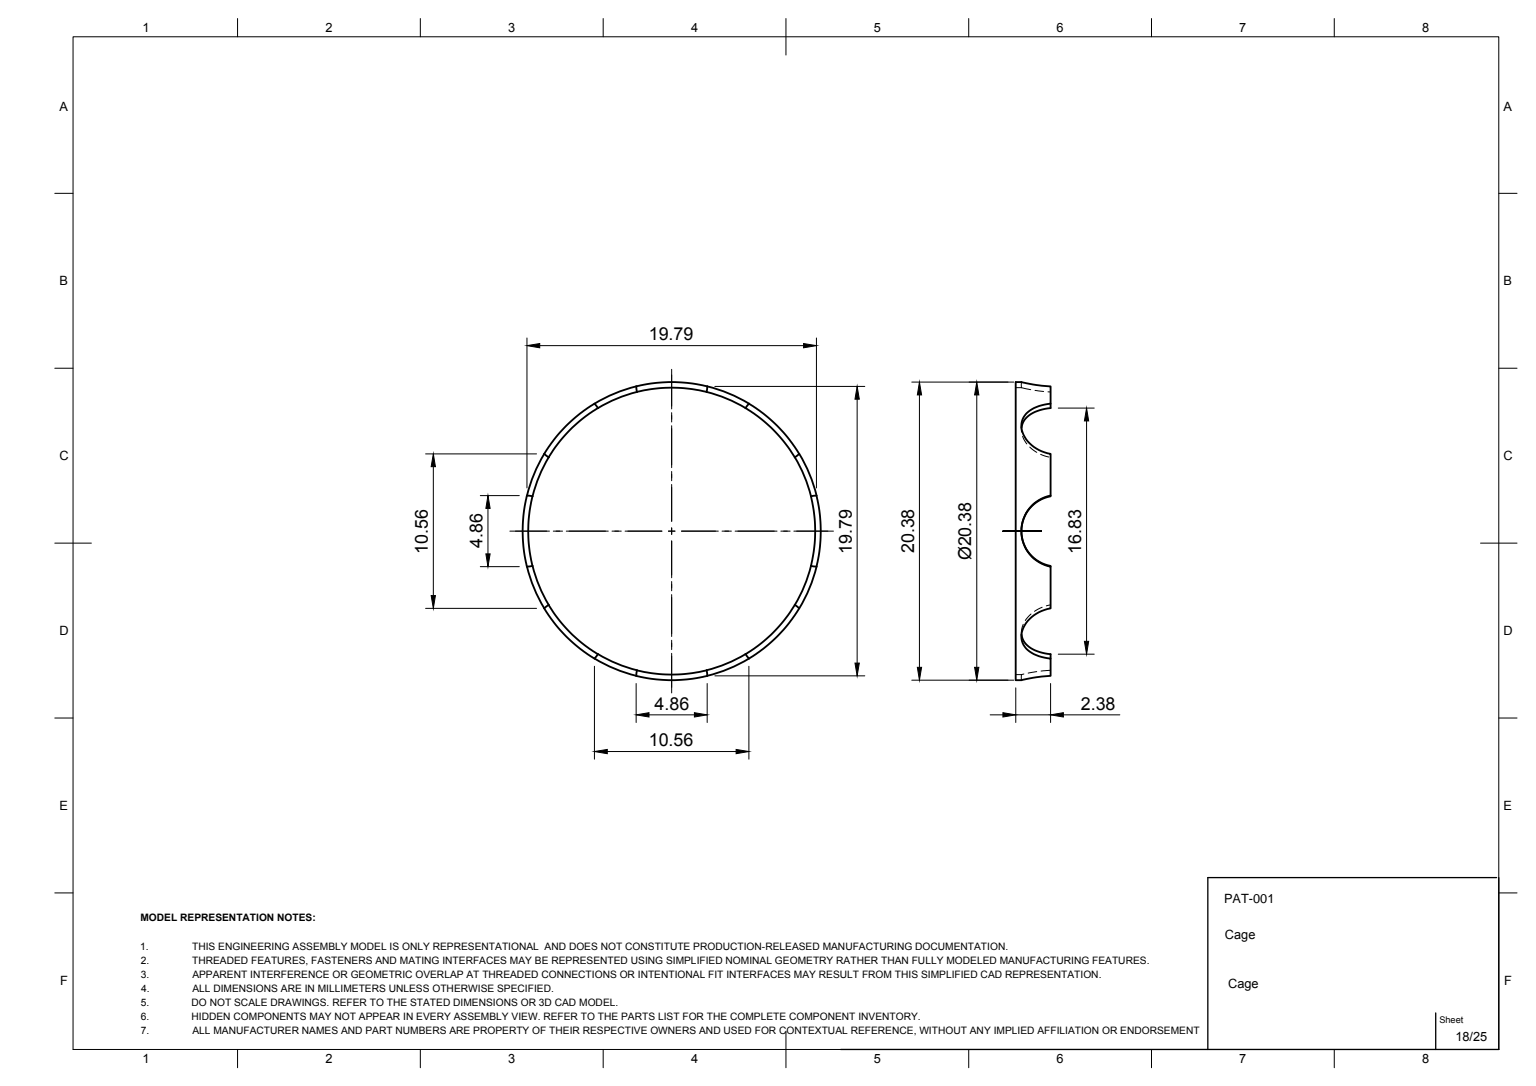
ISO-10303-21;
HEADER;
/* Generated by software containing ST-Developer
 * from STEP Tools, Inc. (www.steptools.com) 
 */

FILE_DESCRIPTION(
/* description */ ('PAT-001'),
/* implementation_level */ '2;1');

FILE_NAME(
/* name */ 'Cage.step',
/* time_stamp */ '2026-10-29T17:07:15-07:00',
/* author */ (''),
/* organization */ (''),
/* preprocessor_version */ 'ST-DEVELOPER v20.2',
/* originating_system */ 'Autodesk Translation Framework v15.17.0.0',
/* authorisation */ '');

FILE_SCHEMA (('AUTOMOTIVE_DESIGN { 1 0 10303 214 3 1 1 }'));
ENDSEC;

DATA;
#10=MECHANICAL_DESIGN_GEOMETRIC_PRESENTATION_REPRESENTATION('',(#388),#9622);
#271=B_SPLINE_CURVE_WITH_KNOTS('',3,(#7915,#7916,#7917,#7918,#7919,#7920,
#7921,#7922,#7923,#7924,#7925,#7926,#7927,#7928,#7929,#7930,#7931,#7932,
#7933,#7934,#7935,#7936),.UNSPECIFIED.,.F.,.F.,(4,2,2,2,2,2,2,2,2,2,4),
(0.0473477652366656,0.126350602536658,0.189525903804987,0.252701205073317,
0.313298422430275,0.373895639787233,0.434492857144191,0.495090074501149,
0.558265375769478,0.621440677037807,0.7004435143378),.UNSPECIFIED.);
#272=B_SPLINE_CURVE_WITH_KNOTS('',3,(#7940,#7941,#7942,#7943,#7944,#7945,
#7946,#7947,#7948,#7949,#7950,#7951,#7952,#7953,#7954,#7955,#7956,#7957,
#7958,#7959,#7960,#7961),.UNSPECIFIED.,.F.,.F.,(4,2,2,2,2,2,2,2,2,2,4),
(0.0464897534940957,0.0852567806515119,0.170513561303024,0.246687263103517,
0.308657850341199,0.370628437578881,0.432599024816563,0.494569612054245,
0.570743313854739,0.656000094506251,0.694767121663666),.UNSPECIFIED.);
#273=B_SPLINE_CURVE_WITH_KNOTS('',3,(#7967,#7968,#7969,#7970,#7971,#7972,
#7973,#7974,#7975,#7976,#7977,#7978,#7979,#7980,#7981,#7982,#7983,#7984,
#7985,#7986,#7987,#7988),.UNSPECIFIED.,.F.,.F.,(4,2,2,2,2,2,2,2,2,2,4),
(0.0464897534940957,0.0852567806515118,0.170513561303024,0.246687263103517,
0.308657850341199,0.370628437578881,0.432599024816563,0.494569612054245,
0.570743313854738,0.65600009450625,0.694767121663666),.UNSPECIFIED.);
#274=B_SPLINE_CURVE_WITH_KNOTS('',3,(#7992,#7993,#7994,#7995,#7996,#7997,
#7998,#7999,#8000,#8001,#8002,#8003,#8004,#8005,#8006,#8007,#8008,#8009,
#8010,#8011,#8012,#8013),.UNSPECIFIED.,.F.,.F.,(4,2,2,2,2,2,2,2,2,2,4),
(0.0464897534940957,0.0852567806515119,0.170513561303024,0.246687263103517,
0.308657850341199,0.370628437578881,0.432599024816563,0.494569612054245,
0.570743313854739,0.656000094506251,0.694767121663666),.UNSPECIFIED.);
#275=B_SPLINE_CURVE_WITH_KNOTS('',3,(#8017,#8018,#8019,#8020,#8021,#8022,
#8023,#8024,#8025,#8026,#8027,#8028),.UNSPECIFIED.,.F.,.F.,(4,2,2,2,2,4),
(0.0464897534940957,0.0852567806515119,0.170513561303024,0.246687263103517,
0.308657850341199,0.370628437578881),.UNSPECIFIED.);
#276=B_SPLINE_CURVE_WITH_KNOTS('',3,(#8033,#8034,#8035,#8036,#8037,#8038,
#8039,#8040,#8041,#8042,#8043,#8044),.UNSPECIFIED.,.F.,.F.,(4,2,2,2,2,4),
(0.370628437578881,0.432599024816563,0.494569612054245,0.570743313854738,
0.65600009450625,0.694767121663666),.UNSPECIFIED.);
#277=B_SPLINE_CURVE_WITH_KNOTS('',3,(#8048,#8049,#8050,#8051,#8052,#8053,
#8054,#8055,#8056,#8057,#8058,#8059,#8060,#8061,#8062,#8063,#8064,#8065,
#8066,#8067,#8068,#8069),.UNSPECIFIED.,.F.,.F.,(4,2,2,2,2,2,2,2,2,2,4),
(0.0464897534940957,0.0852567806515121,0.170513561303024,0.246687263103518,
0.308657850341199,0.370628437578881,0.432599024816563,0.494569612054245,
0.570743313854738,0.65600009450625,0.694767121663666),.UNSPECIFIED.);
#278=B_SPLINE_CURVE_WITH_KNOTS('',3,(#8073,#8074,#8075,#8076,#8077,#8078,
#8079,#8080,#8081,#8082,#8083,#8084,#8085,#8086,#8087,#8088,#8089,#8090,
#8091,#8092,#8093,#8094),.UNSPECIFIED.,.F.,.F.,(4,2,2,2,2,2,2,2,2,2,4),
(0.0464897534940957,0.0852567806515119,0.170513561303024,0.246687263103517,
0.308657850341199,0.370628437578881,0.432599024816563,0.494569612054245,
0.570743313854738,0.65600009450625,0.694767121663667),.UNSPECIFIED.);
#279=B_SPLINE_CURVE_WITH_KNOTS('',3,(#8098,#8099,#8100,#8101,#8102,#8103,
#8104,#8105,#8106,#8107,#8108,#8109,#8110,#8111,#8112,#8113,#8114,#8115,
#8116,#8117,#8118,#8119),.UNSPECIFIED.,.F.,.F.,(4,2,2,2,2,2,2,2,2,2,4),
(0.0464897534940957,0.0852567806515119,0.170513561303024,0.246687263103517,
0.308657850341199,0.370628437578881,0.432599024816563,0.494569612054245,
0.570743313854738,0.65600009450625,0.694767121663666),.UNSPECIFIED.);
#280=B_SPLINE_CURVE_WITH_KNOTS('',3,(#8123,#8124,#8125,#8126,#8127,#8128,
#8129,#8130,#8131,#8132,#8133,#8134,#8135,#8136,#8137,#8138,#8139,#8140,
#8141,#8142,#8143,#8144),.UNSPECIFIED.,.F.,.F.,(4,2,2,2,2,2,2,2,2,2,4),
(0.0464897534940957,0.0852567806515119,0.170513561303024,0.246687263103517,
0.308657850341199,0.370628437578881,0.432599024816563,0.494569612054245,
0.570743313854739,0.656000094506251,0.694767121663667),.UNSPECIFIED.);
#281=B_SPLINE_CURVE_WITH_KNOTS('',3,(#8152,#8153,#8154,#8155,#8156,#8157,
#8158,#8159,#8160,#8161,#8162,#8163,#8164,#8165,#8166,#8167,#8168,#8169,
#8170,#8171,#8172,#8173),.UNSPECIFIED.,.F.,.F.,(4,2,2,2,2,2,2,2,2,2,4),
(0.0473477652366656,0.126350602536658,0.189525903804987,0.252701205073316,
0.313298422430274,0.373895639787232,0.434492857144191,0.495090074501149,
0.558265375769478,0.621440677037807,0.7004435143378),.UNSPECIFIED.);
#282=B_SPLINE_CURVE_WITH_KNOTS('',3,(#8181,#8182,#8183,#8184,#8185,#8186,
#8187,#8188,#8189,#8190,#8191,#8192,#8193,#8194,#8195,#8196,#8197,#8198,
#8199,#8200,#8201,#8202),.UNSPECIFIED.,.F.,.F.,(4,2,2,2,2,2,2,2,2,2,4),
(0.0473477652366656,0.126350602536658,0.189525903804987,0.252701205073317,
0.313298422430275,0.373895639787233,0.434492857144191,0.495090074501149,
0.558265375769478,0.621440677037807,0.7004435143378),.UNSPECIFIED.);
#283=B_SPLINE_CURVE_WITH_KNOTS('',3,(#8211,#8212,#8213,#8214,#8215,#8216,
#8217,#8218,#8219,#8220,#8221,#8222),.UNSPECIFIED.,.F.,.F.,(4,2,2,2,2,4),
(0.0473477652366656,0.126350602536658,0.189525903804987,0.252701205073316,
0.313298422430275,0.373895639787233),.UNSPECIFIED.);
#284=B_SPLINE_CURVE_WITH_KNOTS('',3,(#8224,#8225,#8226,#8227,#8228,#8229,
#8230,#8231,#8232,#8233,#8234,#8235),.UNSPECIFIED.,.F.,.F.,(4,2,2,2,2,4),
(0.373895639787233,0.434492857144191,0.495090074501149,0.558265375769478,
0.621440677037807,0.7004435143378),.UNSPECIFIED.);
#285=B_SPLINE_CURVE_WITH_KNOTS('',3,(#8242,#8243,#8244,#8245,#8246,#8247,
#8248,#8249,#8250,#8251,#8252,#8253,#8254,#8255,#8256,#8257,#8258,#8259,
#8260,#8261,#8262,#8263),.UNSPECIFIED.,.F.,.F.,(4,2,2,2,2,2,2,2,2,2,4),
(0.0473477652366656,0.126350602536658,0.189525903804987,0.252701205073316,
0.313298422430275,0.373895639787233,0.434492857144191,0.495090074501149,
0.558265375769478,0.621440677037807,0.7004435143378),.UNSPECIFIED.);
#286=B_SPLINE_CURVE_WITH_KNOTS('',3,(#8271,#8272,#8273,#8274,#8275,#8276,
#8277,#8278,#8279,#8280,#8281,#8282,#8283,#8284,#8285,#8286,#8287,#8288,
#8289,#8290,#8291,#8292),.UNSPECIFIED.,.F.,.F.,(4,2,2,2,2,2,2,2,2,2,4),
(0.0473477652366656,0.126350602536658,0.189525903804987,0.252701205073317,
0.313298422430275,0.373895639787233,0.434492857144191,0.495090074501149,
0.558265375769478,0.621440677037807,0.7004435143378),.UNSPECIFIED.);
#287=B_SPLINE_CURVE_WITH_KNOTS('',3,(#8300,#8301,#8302,#8303,#8304,#8305,
#8306,#8307,#8308,#8309,#8310,#8311,#8312,#8313,#8314,#8315,#8316,#8317,
#8318,#8319,#8320,#8321),.UNSPECIFIED.,.F.,.F.,(4,2,2,2,2,2,2,2,2,2,4),
(0.0473477652366656,0.126350602536658,0.189525903804987,0.252701205073316,
0.313298422430275,0.373895639787233,0.434492857144191,0.495090074501149,
0.558265375769478,0.621440677037807,0.7004435143378),.UNSPECIFIED.);
#288=B_SPLINE_CURVE_WITH_KNOTS('',3,(#8330,#8331,#8332,#8333,#8334,#8335,
#8336,#8337,#8338,#8339,#8340,#8341,#8342,#8343,#8344,#8345,#8346,#8347,
#8348,#8349,#8350,#8351),.UNSPECIFIED.,.F.,.F.,(4,2,2,2,2,2,2,2,2,2,4),
(0.0473477652366656,0.126350602536658,0.189525903804987,0.252701205073317,
0.313298422430275,0.373895639787233,0.434492857144191,0.495090074501149,
0.558265375769478,0.621440677037807,0.7004435143378),.UNSPECIFIED.);
#297=SPHERICAL_SURFACE('',#5628,0.247676);
#298=SPHERICAL_SURFACE('',#5644,0.247676);
#299=SPHERICAL_SURFACE('',#5649,0.247676);
#300=SPHERICAL_SURFACE('',#5654,0.247676);
#301=SPHERICAL_SURFACE('',#5659,0.247676);
#302=SPHERICAL_SURFACE('',#5664,0.247676);
#303=SPHERICAL_SURFACE('',#5669,0.247676);
#304=SPHERICAL_SURFACE('',#5677,0.247676);
#331=SHAPE_REPRESENTATION_RELATIONSHIP('SRR','None',#9755,#356);
#356=ADVANCED_BREP_SHAPE_REPRESENTATION('',(#421),#9604);
#388=STYLED_ITEM('',(#9962),#421);
#421=MANIFOLD_SOLID_BREP('Continuous crown cage',#5213);
#453=FACE_BOUND('',#1096,.T.);
#546=PLANE('',#5641);
#547=PLANE('',#5646);
#548=PLANE('',#5651);
#549=PLANE('',#5656);
#550=PLANE('',#5661);
#551=PLANE('',#5666);
#552=PLANE('',#5675);
#553=PLANE('',#5679);
#554=PLANE('',#5680);
#766=FACE_OUTER_BOUND('',#1078,.T.);
#767=FACE_OUTER_BOUND('',#1079,.T.);
#768=FACE_OUTER_BOUND('',#1080,.T.);
#769=FACE_OUTER_BOUND('',#1081,.T.);
#770=FACE_OUTER_BOUND('',#1082,.T.);
#771=FACE_OUTER_BOUND('',#1083,.T.);
#772=FACE_OUTER_BOUND('',#1084,.T.);
#773=FACE_OUTER_BOUND('',#1085,.T.);
#774=FACE_OUTER_BOUND('',#1086,.T.);
#775=FACE_OUTER_BOUND('',#1087,.T.);
#776=FACE_OUTER_BOUND('',#1088,.T.);
#777=FACE_OUTER_BOUND('',#1089,.T.);
#778=FACE_OUTER_BOUND('',#1090,.T.);
#779=FACE_OUTER_BOUND('',#1091,.T.);
#780=FACE_OUTER_BOUND('',#1092,.T.);
#781=FACE_OUTER_BOUND('',#1093,.T.);
#782=FACE_OUTER_BOUND('',#1094,.T.);
#783=FACE_OUTER_BOUND('',#1095,.T.);
#784=FACE_OUTER_BOUND('',#1097,.T.);
#1078=EDGE_LOOP('',(#3675,#3676,#3677,#3678));
#1079=EDGE_LOOP('',(#3679,#3680,#3681,#3682,#3683,#3684,#3685,#3686,#3687,
#3688,#3689,#3690,#3691,#3692,#3693,#3694,#3695,#3696,#3697,#3698));
#1080=EDGE_LOOP('',(#3699,#3700,#3701,#3702));
#1081=EDGE_LOOP('',(#3703,#3704,#3705,#3706));
#1082=EDGE_LOOP('',(#3707,#3708,#3709,#3710));
#1083=EDGE_LOOP('',(#3711,#3712,#3713,#3714));
#1084=EDGE_LOOP('',(#3715,#3716,#3717,#3718));
#1085=EDGE_LOOP('',(#3719,#3720,#3721,#3722,#3723,#3724));
#1086=EDGE_LOOP('',(#3725,#3726,#3727,#3728));
#1087=EDGE_LOOP('',(#3729,#3730,#3731,#3732));
#1088=EDGE_LOOP('',(#3733,#3734,#3735,#3736));
#1089=EDGE_LOOP('',(#3737,#3738,#3739,#3740));
#1090=EDGE_LOOP('',(#3741,#3742,#3743,#3744));
#1091=EDGE_LOOP('',(#3745,#3746,#3747,#3748));
#1092=EDGE_LOOP('',(#3749,#3750,#3751,#3752,#3753,#3754,#3755,#3756,#3757,
#3758,#3759,#3760,#3761,#3762,#3763,#3764,#3765,#3766,#3767,#3768));
#1093=EDGE_LOOP('',(#3769,#3770,#3771,#3772));
#1094=EDGE_LOOP('',(#3773,#3774,#3775,#3776));
#1095=EDGE_LOOP('',(#3777));
#1096=EDGE_LOOP('',(#3778));
#1097=EDGE_LOOP('',(#3779,#3780,#3781,#3782));
#1421=LINE('',#8030,#1826);
#1422=LINE('',#8326,#1827);
#1826=VECTOR('',#6382,1.019052);
#1827=VECTOR('',#6459,0.980948);
#2264=CIRCLE('',#5629,0.243053047864041);
#2265=CIRCLE('',#5630,0.243053047864041);
#2266=CIRCLE('',#5632,1.019052);
#2267=CIRCLE('',#5633,1.019052);
#2268=CIRCLE('',#5634,1.019052);
#2269=CIRCLE('',#5635,1.019052);
#2270=CIRCLE('',#5636,1.019052);
#2271=CIRCLE('',#5637,1.019052);
#2272=CIRCLE('',#5638,1.019052);
#2273=CIRCLE('',#5639,1.019052);
#2274=CIRCLE('',#5640,1.019052);
#2275=CIRCLE('',#5642,0.980948);
#2276=CIRCLE('',#5643,0.243053047864041);
#2277=CIRCLE('',#5645,0.243053047864041);
#2278=CIRCLE('',#5647,0.980948);
#2279=CIRCLE('',#5648,0.243053047864041);
#2280=CIRCLE('',#5650,0.243053047864041);
#2281=CIRCLE('',#5652,0.980948);
#2282=CIRCLE('',#5653,0.243053047864041);
#2283=CIRCLE('',#5655,0.243053047864041);
#2284=CIRCLE('',#5657,0.980948);
#2285=CIRCLE('',#5658,0.243053047864041);
#2286=CIRCLE('',#5660,0.243053047864041);
#2287=CIRCLE('',#5662,0.980948);
#2288=CIRCLE('',#5663,0.243053047864041);
#2289=CIRCLE('',#5665,0.243053047864041);
#2290=CIRCLE('',#5667,0.980948);
#2291=CIRCLE('',#5668,0.243053047864041);
#2292=CIRCLE('',#5670,0.243053047864041);
#2293=CIRCLE('',#5672,0.980948);
#2294=CIRCLE('',#5673,0.980948);
#2295=CIRCLE('',#5674,0.980948);
#2296=CIRCLE('',#5676,0.243053047864041);
#2297=CIRCLE('',#5678,0.243053047864041);
#2482=VERTEX_POINT('',#7913);
#2483=VERTEX_POINT('',#7914);
#2484=VERTEX_POINT('',#7937);
#2485=VERTEX_POINT('',#7939);
#2486=VERTEX_POINT('',#7964);
#2487=VERTEX_POINT('',#7966);
#2488=VERTEX_POINT('',#7989);
#2489=VERTEX_POINT('',#7991);
#2490=VERTEX_POINT('',#8014);
#2491=VERTEX_POINT('',#8016);
#2492=VERTEX_POINT('',#8029);
#2493=VERTEX_POINT('',#8032);
#2494=VERTEX_POINT('',#8045);
#2495=VERTEX_POINT('',#8047);
#2496=VERTEX_POINT('',#8070);
#2497=VERTEX_POINT('',#8072);
#2498=VERTEX_POINT('',#8095);
#2499=VERTEX_POINT('',#8097);
#2500=VERTEX_POINT('',#8120);
#2501=VERTEX_POINT('',#8122);
#2502=VERTEX_POINT('',#8147);
#2503=VERTEX_POINT('',#8151);
#2504=VERTEX_POINT('',#8176);
#2505=VERTEX_POINT('',#8180);
#2506=VERTEX_POINT('',#8205);
#2507=VERTEX_POINT('',#8209);
#2508=VERTEX_POINT('',#8210);
#2509=VERTEX_POINT('',#8237);
#2510=VERTEX_POINT('',#8241);
#2511=VERTEX_POINT('',#8266);
#2512=VERTEX_POINT('',#8270);
#2513=VERTEX_POINT('',#8295);
#2514=VERTEX_POINT('',#8299);
#2515=VERTEX_POINT('',#8324);
#2516=VERTEX_POINT('',#8327);
#2517=VERTEX_POINT('',#8329);
#2941=EDGE_CURVE('',#2482,#2483,#271,.T.);
#2942=EDGE_CURVE('',#2484,#2482,#2264,.T.);
#2943=EDGE_CURVE('',#2485,#2484,#272,.T.);
#2944=EDGE_CURVE('',#2483,#2485,#2265,.T.);
#2945=EDGE_CURVE('',#2486,#2484,#2266,.T.);
#2946=EDGE_CURVE('',#2486,#2487,#273,.T.);
#2947=EDGE_CURVE('',#2488,#2487,#2267,.T.);
#2948=EDGE_CURVE('',#2488,#2489,#274,.T.);
#2949=EDGE_CURVE('',#2490,#2489,#2268,.T.);
#2950=EDGE_CURVE('',#2490,#2491,#275,.T.);
#2951=EDGE_CURVE('',#2491,#2492,#1421,.T.);
#2952=EDGE_CURVE('',#2492,#2492,#2269,.T.);
#2953=EDGE_CURVE('',#2491,#2493,#276,.T.);
#2954=EDGE_CURVE('',#2494,#2493,#2270,.T.);
#2955=EDGE_CURVE('',#2494,#2495,#277,.T.);
#2956=EDGE_CURVE('',#2496,#2495,#2271,.T.);
#2957=EDGE_CURVE('',#2496,#2497,#278,.T.);
#2958=EDGE_CURVE('',#2498,#2497,#2272,.T.);
#2959=EDGE_CURVE('',#2498,#2499,#279,.T.);
#2960=EDGE_CURVE('',#2500,#2499,#2273,.T.);
#2961=EDGE_CURVE('',#2500,#2501,#280,.T.);
#2962=EDGE_CURVE('',#2485,#2501,#2274,.T.);
#2963=EDGE_CURVE('',#2482,#2502,#2275,.T.);
#2964=EDGE_CURVE('',#2502,#2486,#2276,.T.);
#2965=EDGE_CURVE('',#2503,#2502,#281,.T.);
#2966=EDGE_CURVE('',#2487,#2503,#2277,.T.);
#2967=EDGE_CURVE('',#2503,#2504,#2278,.T.);
#2968=EDGE_CURVE('',#2504,#2488,#2279,.T.);
#2969=EDGE_CURVE('',#2505,#2504,#282,.T.);
#2970=EDGE_CURVE('',#2489,#2505,#2280,.T.);
#2971=EDGE_CURVE('',#2505,#2506,#2281,.T.);
#2972=EDGE_CURVE('',#2506,#2490,#2282,.T.);
#2973=EDGE_CURVE('',#2507,#2508,#283,.T.);
#2974=EDGE_CURVE('',#2493,#2507,#2283,.T.);
#2975=EDGE_CURVE('',#2508,#2506,#284,.T.);
#2976=EDGE_CURVE('',#2507,#2509,#2284,.T.);
#2977=EDGE_CURVE('',#2509,#2494,#2285,.T.);
#2978=EDGE_CURVE('',#2510,#2509,#285,.T.);
#2979=EDGE_CURVE('',#2495,#2510,#2286,.T.);
#2980=EDGE_CURVE('',#2510,#2511,#2287,.T.);
#2981=EDGE_CURVE('',#2511,#2496,#2288,.T.);
#2982=EDGE_CURVE('',#2512,#2511,#286,.T.);
#2983=EDGE_CURVE('',#2497,#2512,#2289,.T.);
#2984=EDGE_CURVE('',#2512,#2513,#2290,.T.);
#2985=EDGE_CURVE('',#2513,#2498,#2291,.T.);
#2986=EDGE_CURVE('',#2514,#2513,#287,.T.);
#2987=EDGE_CURVE('',#2499,#2514,#2292,.T.);
#2988=EDGE_CURVE('',#2515,#2515,#2293,.T.);
#2989=EDGE_CURVE('',#2515,#2508,#1422,.T.);
#2990=EDGE_CURVE('',#2516,#2483,#2294,.T.);
#2991=EDGE_CURVE('',#2516,#2517,#288,.T.);
#2992=EDGE_CURVE('',#2514,#2517,#2295,.T.);
#2993=EDGE_CURVE('',#2501,#2516,#2296,.T.);
#2994=EDGE_CURVE('',#2517,#2500,#2297,.T.);
#3675=ORIENTED_EDGE('',*,*,#2941,.F.);
#3676=ORIENTED_EDGE('',*,*,#2942,.F.);
#3677=ORIENTED_EDGE('',*,*,#2943,.F.);
#3678=ORIENTED_EDGE('',*,*,#2944,.F.);
#3679=ORIENTED_EDGE('',*,*,#2943,.T.);
#3680=ORIENTED_EDGE('',*,*,#2945,.F.);
#3681=ORIENTED_EDGE('',*,*,#2946,.T.);
#3682=ORIENTED_EDGE('',*,*,#2947,.F.);
#3683=ORIENTED_EDGE('',*,*,#2948,.T.);
#3684=ORIENTED_EDGE('',*,*,#2949,.F.);
#3685=ORIENTED_EDGE('',*,*,#2950,.T.);
#3686=ORIENTED_EDGE('',*,*,#2951,.T.);
#3687=ORIENTED_EDGE('',*,*,#2952,.F.);
#3688=ORIENTED_EDGE('',*,*,#2951,.F.);
#3689=ORIENTED_EDGE('',*,*,#2953,.T.);
#3690=ORIENTED_EDGE('',*,*,#2954,.F.);
#3691=ORIENTED_EDGE('',*,*,#2955,.T.);
#3692=ORIENTED_EDGE('',*,*,#2956,.F.);
#3693=ORIENTED_EDGE('',*,*,#2957,.T.);
#3694=ORIENTED_EDGE('',*,*,#2958,.F.);
#3695=ORIENTED_EDGE('',*,*,#2959,.T.);
#3696=ORIENTED_EDGE('',*,*,#2960,.F.);
#3697=ORIENTED_EDGE('',*,*,#2961,.T.);
#3698=ORIENTED_EDGE('',*,*,#2962,.F.);
#3699=ORIENTED_EDGE('',*,*,#2942,.T.);
#3700=ORIENTED_EDGE('',*,*,#2963,.T.);
#3701=ORIENTED_EDGE('',*,*,#2964,.T.);
#3702=ORIENTED_EDGE('',*,*,#2945,.T.);
#3703=ORIENTED_EDGE('',*,*,#2965,.F.);
#3704=ORIENTED_EDGE('',*,*,#2966,.F.);
#3705=ORIENTED_EDGE('',*,*,#2946,.F.);
#3706=ORIENTED_EDGE('',*,*,#2964,.F.);
#3707=ORIENTED_EDGE('',*,*,#2966,.T.);
#3708=ORIENTED_EDGE('',*,*,#2967,.T.);
#3709=ORIENTED_EDGE('',*,*,#2968,.T.);
#3710=ORIENTED_EDGE('',*,*,#2947,.T.);
#3711=ORIENTED_EDGE('',*,*,#2969,.F.);
#3712=ORIENTED_EDGE('',*,*,#2970,.F.);
#3713=ORIENTED_EDGE('',*,*,#2948,.F.);
#3714=ORIENTED_EDGE('',*,*,#2968,.F.);
#3715=ORIENTED_EDGE('',*,*,#2970,.T.);
#3716=ORIENTED_EDGE('',*,*,#2971,.T.);
#3717=ORIENTED_EDGE('',*,*,#2972,.T.);
#3718=ORIENTED_EDGE('',*,*,#2949,.T.);
#3719=ORIENTED_EDGE('',*,*,#2973,.F.);
#3720=ORIENTED_EDGE('',*,*,#2974,.F.);
#3721=ORIENTED_EDGE('',*,*,#2953,.F.);
#3722=ORIENTED_EDGE('',*,*,#2950,.F.);
#3723=ORIENTED_EDGE('',*,*,#2972,.F.);
#3724=ORIENTED_EDGE('',*,*,#2975,.F.);
#3725=ORIENTED_EDGE('',*,*,#2974,.T.);
#3726=ORIENTED_EDGE('',*,*,#2976,.T.);
#3727=ORIENTED_EDGE('',*,*,#2977,.T.);
#3728=ORIENTED_EDGE('',*,*,#2954,.T.);
#3729=ORIENTED_EDGE('',*,*,#2978,.F.);
#3730=ORIENTED_EDGE('',*,*,#2979,.F.);
#3731=ORIENTED_EDGE('',*,*,#2955,.F.);
#3732=ORIENTED_EDGE('',*,*,#2977,.F.);
#3733=ORIENTED_EDGE('',*,*,#2979,.T.);
#3734=ORIENTED_EDGE('',*,*,#2980,.T.);
#3735=ORIENTED_EDGE('',*,*,#2981,.T.);
#3736=ORIENTED_EDGE('',*,*,#2956,.T.);
#3737=ORIENTED_EDGE('',*,*,#2982,.F.);
#3738=ORIENTED_EDGE('',*,*,#2983,.F.);
#3739=ORIENTED_EDGE('',*,*,#2957,.F.);
#3740=ORIENTED_EDGE('',*,*,#2981,.F.);
#3741=ORIENTED_EDGE('',*,*,#2983,.T.);
#3742=ORIENTED_EDGE('',*,*,#2984,.T.);
#3743=ORIENTED_EDGE('',*,*,#2985,.T.);
#3744=ORIENTED_EDGE('',*,*,#2958,.T.);
#3745=ORIENTED_EDGE('',*,*,#2959,.F.);
#3746=ORIENTED_EDGE('',*,*,#2985,.F.);
#3747=ORIENTED_EDGE('',*,*,#2986,.F.);
#3748=ORIENTED_EDGE('',*,*,#2987,.F.);
#3749=ORIENTED_EDGE('',*,*,#2988,.F.);
#3750=ORIENTED_EDGE('',*,*,#2989,.T.);
#3751=ORIENTED_EDGE('',*,*,#2975,.T.);
#3752=ORIENTED_EDGE('',*,*,#2971,.F.);
#3753=ORIENTED_EDGE('',*,*,#2969,.T.);
#3754=ORIENTED_EDGE('',*,*,#2967,.F.);
#3755=ORIENTED_EDGE('',*,*,#2965,.T.);
#3756=ORIENTED_EDGE('',*,*,#2963,.F.);
#3757=ORIENTED_EDGE('',*,*,#2941,.T.);
#3758=ORIENTED_EDGE('',*,*,#2990,.F.);
#3759=ORIENTED_EDGE('',*,*,#2991,.T.);
#3760=ORIENTED_EDGE('',*,*,#2992,.F.);
#3761=ORIENTED_EDGE('',*,*,#2986,.T.);
#3762=ORIENTED_EDGE('',*,*,#2984,.F.);
#3763=ORIENTED_EDGE('',*,*,#2982,.T.);
#3764=ORIENTED_EDGE('',*,*,#2980,.F.);
#3765=ORIENTED_EDGE('',*,*,#2978,.T.);
#3766=ORIENTED_EDGE('',*,*,#2976,.F.);
#3767=ORIENTED_EDGE('',*,*,#2973,.T.);
#3768=ORIENTED_EDGE('',*,*,#2989,.F.);
#3769=ORIENTED_EDGE('',*,*,#2944,.T.);
#3770=ORIENTED_EDGE('',*,*,#2962,.T.);
#3771=ORIENTED_EDGE('',*,*,#2993,.T.);
#3772=ORIENTED_EDGE('',*,*,#2990,.T.);
#3773=ORIENTED_EDGE('',*,*,#2961,.F.);
#3774=ORIENTED_EDGE('',*,*,#2994,.F.);
#3775=ORIENTED_EDGE('',*,*,#2991,.F.);
#3776=ORIENTED_EDGE('',*,*,#2993,.F.);
#3777=ORIENTED_EDGE('',*,*,#2952,.T.);
#3778=ORIENTED_EDGE('',*,*,#2988,.T.);
#3779=ORIENTED_EDGE('',*,*,#2987,.T.);
#3780=ORIENTED_EDGE('',*,*,#2992,.T.);
#3781=ORIENTED_EDGE('',*,*,#2994,.T.);
#3782=ORIENTED_EDGE('',*,*,#2960,.T.);
#4846=CYLINDRICAL_SURFACE('',#5631,1.019052);
#4847=CYLINDRICAL_SURFACE('',#5671,0.980948);
#4953=ADVANCED_FACE('',(#766),#297,.F.);
#4954=ADVANCED_FACE('',(#767),#4846,.T.);
#4955=ADVANCED_FACE('',(#768),#546,.T.);
#4956=ADVANCED_FACE('',(#769),#298,.F.);
#4957=ADVANCED_FACE('',(#770),#547,.T.);
#4958=ADVANCED_FACE('',(#771),#299,.F.);
#4959=ADVANCED_FACE('',(#772),#548,.T.);
#4960=ADVANCED_FACE('',(#773),#300,.F.);
#4961=ADVANCED_FACE('',(#774),#549,.T.);
#4962=ADVANCED_FACE('',(#775),#301,.F.);
#4963=ADVANCED_FACE('',(#776),#550,.T.);
#4964=ADVANCED_FACE('',(#777),#302,.F.);
#4965=ADVANCED_FACE('',(#778),#551,.T.);
#4966=ADVANCED_FACE('',(#779),#303,.F.);
#4967=ADVANCED_FACE('',(#780),#4847,.F.);
#4968=ADVANCED_FACE('',(#781),#552,.T.);
#4969=ADVANCED_FACE('',(#782),#304,.F.);
#4970=ADVANCED_FACE('',(#783,#453),#553,.T.);
#4971=ADVANCED_FACE('',(#784),#554,.T.);
#5213=CLOSED_SHELL('',(#4953,#4954,#4955,#4956,#4957,#4958,#4959,#4960,
#4961,#4962,#4963,#4964,#4965,#4966,#4967,#4968,#4969,#4970,#4971));
#5627=AXIS2_PLACEMENT_3D('',#7911,#6366,#6367);
#5628=AXIS2_PLACEMENT_3D('',#7912,#6368,#6369);
#5629=AXIS2_PLACEMENT_3D('',#7938,#6370,#6371);
#5630=AXIS2_PLACEMENT_3D('',#7962,#6372,#6373);
#5631=AXIS2_PLACEMENT_3D('',#7963,#6374,#6375);
#5632=AXIS2_PLACEMENT_3D('',#7965,#6376,#6377);
#5633=AXIS2_PLACEMENT_3D('',#7990,#6378,#6379);
#5634=AXIS2_PLACEMENT_3D('',#8015,#6380,#6381);
#5635=AXIS2_PLACEMENT_3D('',#8031,#6383,#6384);
#5636=AXIS2_PLACEMENT_3D('',#8046,#6385,#6386);
#5637=AXIS2_PLACEMENT_3D('',#8071,#6387,#6388);
#5638=AXIS2_PLACEMENT_3D('',#8096,#6389,#6390);
#5639=AXIS2_PLACEMENT_3D('',#8121,#6391,#6392);
#5640=AXIS2_PLACEMENT_3D('',#8145,#6393,#6394);
#5641=AXIS2_PLACEMENT_3D('',#8146,#6395,#6396);
#5642=AXIS2_PLACEMENT_3D('',#8148,#6397,#6398);
#5643=AXIS2_PLACEMENT_3D('',#8149,#6399,#6400);
#5644=AXIS2_PLACEMENT_3D('',#8150,#6401,#6402);
#5645=AXIS2_PLACEMENT_3D('',#8174,#6403,#6404);
#5646=AXIS2_PLACEMENT_3D('',#8175,#6405,#6406);
#5647=AXIS2_PLACEMENT_3D('',#8177,#6407,#6408);
#5648=AXIS2_PLACEMENT_3D('',#8178,#6409,#6410);
#5649=AXIS2_PLACEMENT_3D('',#8179,#6411,#6412);
#5650=AXIS2_PLACEMENT_3D('',#8203,#6413,#6414);
#5651=AXIS2_PLACEMENT_3D('',#8204,#6415,#6416);
#5652=AXIS2_PLACEMENT_3D('',#8206,#6417,#6418);
#5653=AXIS2_PLACEMENT_3D('',#8207,#6419,#6420);
#5654=AXIS2_PLACEMENT_3D('',#8208,#6421,#6422);
#5655=AXIS2_PLACEMENT_3D('',#8223,#6423,#6424);
#5656=AXIS2_PLACEMENT_3D('',#8236,#6425,#6426);
#5657=AXIS2_PLACEMENT_3D('',#8238,#6427,#6428);
#5658=AXIS2_PLACEMENT_3D('',#8239,#6429,#6430);
#5659=AXIS2_PLACEMENT_3D('',#8240,#6431,#6432);
#5660=AXIS2_PLACEMENT_3D('',#8264,#6433,#6434);
#5661=AXIS2_PLACEMENT_3D('',#8265,#6435,#6436);
#5662=AXIS2_PLACEMENT_3D('',#8267,#6437,#6438);
#5663=AXIS2_PLACEMENT_3D('',#8268,#6439,#6440);
#5664=AXIS2_PLACEMENT_3D('',#8269,#6441,#6442);
#5665=AXIS2_PLACEMENT_3D('',#8293,#6443,#6444);
#5666=AXIS2_PLACEMENT_3D('',#8294,#6445,#6446);
#5667=AXIS2_PLACEMENT_3D('',#8296,#6447,#6448);
#5668=AXIS2_PLACEMENT_3D('',#8297,#6449,#6450);
#5669=AXIS2_PLACEMENT_3D('',#8298,#6451,#6452);
#5670=AXIS2_PLACEMENT_3D('',#8322,#6453,#6454);
#5671=AXIS2_PLACEMENT_3D('',#8323,#6455,#6456);
#5672=AXIS2_PLACEMENT_3D('',#8325,#6457,#6458);
#5673=AXIS2_PLACEMENT_3D('',#8328,#6460,#6461);
#5674=AXIS2_PLACEMENT_3D('',#8352,#6462,#6463);
#5675=AXIS2_PLACEMENT_3D('',#8353,#6464,#6465);
#5676=AXIS2_PLACEMENT_3D('',#8354,#6466,#6467);
#5677=AXIS2_PLACEMENT_3D('',#8355,#6468,#6469);
#5678=AXIS2_PLACEMENT_3D('',#8356,#6470,#6471);
#5679=AXIS2_PLACEMENT_3D('',#8357,#6472,#6473);
#5680=AXIS2_PLACEMENT_3D('',#8358,#6474,#6475);
#6366=DIRECTION('axis',(0.,0.,1.));
#6367=DIRECTION('refdir',(1.,0.,0.));
#6368=DIRECTION('center_axis',(0.,0.,1.));
#6369=DIRECTION('ref_axis',(1.,0.,0.));
#6370=DIRECTION('center_axis',(0.,-1.,0.));
#6371=DIRECTION('ref_axis',(0.,0.,-1.));
#6372=DIRECTION('center_axis',(0.,-1.,0.));
#6373=DIRECTION('ref_axis',(0.,0.,-1.));
#6374=DIRECTION('center_axis',(0.,1.,0.));
#6375=DIRECTION('ref_axis',(1.,0.,0.));
#6376=DIRECTION('center_axis',(0.,1.,0.));
#6377=DIRECTION('ref_axis',(1.,0.,0.));
#6378=DIRECTION('center_axis',(0.,1.,0.));
#6379=DIRECTION('ref_axis',(1.,0.,0.));
#6380=DIRECTION('center_axis',(0.,1.,0.));
#6381=DIRECTION('ref_axis',(1.,0.,0.));
#6382=DIRECTION('',(0.,-1.,0.));
#6383=DIRECTION('center_axis',(0.,-1.,0.));
#6384=DIRECTION('ref_axis',(1.,0.,0.));
#6385=DIRECTION('center_axis',(0.,1.,0.));
#6386=DIRECTION('ref_axis',(1.,0.,0.));
#6387=DIRECTION('center_axis',(0.,1.,0.));
#6388=DIRECTION('ref_axis',(1.,0.,0.));
#6389=DIRECTION('center_axis',(0.,1.,0.));
#6390=DIRECTION('ref_axis',(1.,0.,0.));
#6391=DIRECTION('center_axis',(0.,1.,0.));
#6392=DIRECTION('ref_axis',(1.,0.,0.));
#6393=DIRECTION('center_axis',(0.,1.,0.));
#6394=DIRECTION('ref_axis',(1.,0.,0.));
#6395=DIRECTION('center_axis',(0.,1.,0.));
#6396=DIRECTION('ref_axis',(1.,0.,0.));
#6397=DIRECTION('center_axis',(0.,-1.,0.));
#6398=DIRECTION('ref_axis',(1.,0.,0.));
#6399=DIRECTION('center_axis',(0.,-1.,0.));
#6400=DIRECTION('ref_axis',(0.,0.,-1.));
#6401=DIRECTION('center_axis',(6.12323399573677E-17,0.,1.));
#6402=DIRECTION('ref_axis',(1.,0.,0.));
#6403=DIRECTION('center_axis',(0.,-1.,0.));
#6404=DIRECTION('ref_axis',(0.,0.,-1.));
#6405=DIRECTION('center_axis',(0.,1.,0.));
#6406=DIRECTION('ref_axis',(1.,0.,0.));
#6407=DIRECTION('center_axis',(0.,-1.,0.));
#6408=DIRECTION('ref_axis',(1.,0.,0.));
#6409=DIRECTION('center_axis',(0.,-1.,0.));
#6410=DIRECTION('ref_axis',(0.,0.,-1.));
#6411=DIRECTION('center_axis',(0.,0.,1.));
#6412=DIRECTION('ref_axis',(1.,0.,0.));
#6413=DIRECTION('center_axis',(0.,-1.,0.));
#6414=DIRECTION('ref_axis',(0.,0.,-1.));
#6415=DIRECTION('center_axis',(0.,1.,0.));
#6416=DIRECTION('ref_axis',(1.,0.,0.));
#6417=DIRECTION('center_axis',(0.,-1.,0.));
#6418=DIRECTION('ref_axis',(1.,0.,0.));
#6419=DIRECTION('center_axis',(0.,-1.,0.));
#6420=DIRECTION('ref_axis',(0.,0.,-1.));
#6421=DIRECTION('center_axis',(0.,0.,1.));
#6422=DIRECTION('ref_axis',(1.,0.,0.));
#6423=DIRECTION('center_axis',(0.,-1.,0.));
#6424=DIRECTION('ref_axis',(0.,0.,-1.));
#6425=DIRECTION('center_axis',(0.,1.,0.));
#6426=DIRECTION('ref_axis',(1.,0.,0.));
#6427=DIRECTION('center_axis',(0.,-1.,0.));
#6428=DIRECTION('ref_axis',(1.,0.,0.));
#6429=DIRECTION('center_axis',(0.,-1.,0.));
#6430=DIRECTION('ref_axis',(0.,0.,-1.));
#6431=DIRECTION('center_axis',(0.,0.,1.));
#6432=DIRECTION('ref_axis',(1.,0.,0.));
#6433=DIRECTION('center_axis',(0.,-1.,0.));
#6434=DIRECTION('ref_axis',(0.,0.,-1.));
#6435=DIRECTION('center_axis',(0.,1.,0.));
#6436=DIRECTION('ref_axis',(1.,0.,0.));
#6437=DIRECTION('center_axis',(0.,-1.,0.));
#6438=DIRECTION('ref_axis',(1.,0.,0.));
#6439=DIRECTION('center_axis',(0.,-1.,0.));
#6440=DIRECTION('ref_axis',(0.,0.,-1.));
#6441=DIRECTION('center_axis',(6.12323399573676E-17,0.,1.));
#6442=DIRECTION('ref_axis',(1.,0.,0.));
#6443=DIRECTION('center_axis',(0.,-1.,0.));
#6444=DIRECTION('ref_axis',(0.,0.,-1.));
#6445=DIRECTION('center_axis',(0.,1.,0.));
#6446=DIRECTION('ref_axis',(1.,0.,0.));
#6447=DIRECTION('center_axis',(0.,-1.,0.));
#6448=DIRECTION('ref_axis',(1.,0.,0.));
#6449=DIRECTION('center_axis',(0.,-1.,0.));
#6450=DIRECTION('ref_axis',(0.,0.,-1.));
#6451=DIRECTION('center_axis',(0.,0.,1.));
#6452=DIRECTION('ref_axis',(1.,0.,0.));
#6453=DIRECTION('center_axis',(0.,-1.,0.));
#6454=DIRECTION('ref_axis',(0.,0.,-1.));
#6455=DIRECTION('center_axis',(0.,1.,0.));
#6456=DIRECTION('ref_axis',(1.,0.,0.));
#6457=DIRECTION('center_axis',(0.,1.,0.));
#6458=DIRECTION('ref_axis',(1.,0.,0.));
#6459=DIRECTION('',(0.,1.,0.));
#6460=DIRECTION('center_axis',(0.,-1.,0.));
#6461=DIRECTION('ref_axis',(1.,0.,0.));
#6462=DIRECTION('center_axis',(0.,-1.,0.));
#6463=DIRECTION('ref_axis',(1.,0.,0.));
#6464=DIRECTION('center_axis',(0.,1.,0.));
#6465=DIRECTION('ref_axis',(1.,0.,0.));
#6466=DIRECTION('center_axis',(0.,-1.,0.));
#6467=DIRECTION('ref_axis',(0.,0.,-1.));
#6468=DIRECTION('center_axis',(0.,0.,1.));
#6469=DIRECTION('ref_axis',(1.,0.,0.));
#6470=DIRECTION('center_axis',(0.,-1.,0.));
#6471=DIRECTION('ref_axis',(0.,0.,-1.));
#6472=DIRECTION('center_axis',(0.,-1.,0.));
#6473=DIRECTION('ref_axis',(-1.,0.,0.));
#6474=DIRECTION('center_axis',(0.,1.,0.));
#6475=DIRECTION('ref_axis',(1.,0.,0.));
#7911=CARTESIAN_POINT('',(0.,0.,0.));
#7912=CARTESIAN_POINT('Origin',(0.707106781186547,0.,0.707106781186548));
#7913=CARTESIAN_POINT('',(0.504455939115715,-0.04763,0.841298510752802));
#7914=CARTESIAN_POINT('',(0.841298510752802,-0.04763,0.504455939115715));
#7915=CARTESIAN_POINT('Ctrl Pts',(0.504455939115715,-0.04763,0.841298510752802));
#7916=CARTESIAN_POINT('Ctrl Pts',(0.508899795931835,-0.0740444353928835,
0.838633903678357));
#7917=CARTESIAN_POINT('Ctrl Pts',(0.517157748491652,-0.0999305678883309,
0.833661031856294));
#7918=CARTESIAN_POINT('Ctrl Pts',(0.537715343527944,-0.142345102874864,
0.820511285096538));
#7919=CARTESIAN_POINT('Ctrl Pts',(0.548874290046456,-0.159766064500479,
0.813159949759));
#7920=CARTESIAN_POINT('Ctrl Pts',(0.573915184558107,-0.190326085855194,
0.795684265985089));
#7921=CARTESIAN_POINT('Ctrl Pts',(0.587792702767295,-0.203463743702801,
0.78555112003688));
#7922=CARTESIAN_POINT('Ctrl Pts',(0.615966552324775,-0.224161999508995,
0.763642258217233));
#7923=CARTESIAN_POINT('Ctrl Pts',(0.631684198665438,-0.232861760990032,
0.750785745543687));
#7924=CARTESIAN_POINT('Ctrl Pts',(0.663382628119203,-0.244251601209411,
0.722929908501543));
#7925=CARTESIAN_POINT('Ctrl Pts',(0.679352081686668,-0.246942143572133,
0.707917883896095));
#7926=CARTESIAN_POINT('Ctrl Pts',(0.707917883896095,-0.246942143572133,
0.679352081686668));
#7927=CARTESIAN_POINT('Ctrl Pts',(0.722929908501543,-0.244251601209411,
0.663382628119203));
#7928=CARTESIAN_POINT('Ctrl Pts',(0.750785745543687,-0.232861760990032,
0.631684198665439));
#7929=CARTESIAN_POINT('Ctrl Pts',(0.763642258217232,-0.224161999508995,
0.615966552324775));
#7930=CARTESIAN_POINT('Ctrl Pts',(0.78555112003688,-0.203463743702801,0.587792702767295));
#7931=CARTESIAN_POINT('Ctrl Pts',(0.795684265985088,-0.190326085855194,
0.573915184558108));
#7932=CARTESIAN_POINT('Ctrl Pts',(0.813159949759,-0.15976606450048,0.548874290046456));
#7933=CARTESIAN_POINT('Ctrl Pts',(0.820511285096538,-0.142345102874864,
0.537715343527944));
#7934=CARTESIAN_POINT('Ctrl Pts',(0.833661031856294,-0.099930567888331,
0.517157748491653));
#7935=CARTESIAN_POINT('Ctrl Pts',(0.838633903678357,-0.0740444353928835,
0.508899795931835));
#7936=CARTESIAN_POINT('Ctrl Pts',(0.841298510752801,-0.0476299999999999,
0.504455939115715));
#7937=CARTESIAN_POINT('',(0.528110872004958,-0.04763,0.871530771444223));
#7938=CARTESIAN_POINT('Origin',(0.707106781186547,-0.04763,0.707106781186548));
#7939=CARTESIAN_POINT('',(0.871530771444223,-0.04763,0.528110872004959));
#7940=CARTESIAN_POINT('Ctrl Pts',(0.871530771444223,-0.0476300000000001,
0.528110872004958));
#7941=CARTESIAN_POINT('Ctrl Pts',(0.87014664509073,-0.0609922781173483,
0.530395067942936));
#7942=CARTESIAN_POINT('Ctrl Pts',(0.868149331745851,-0.0742967091364493,
0.533674141594226));
#7943=CARTESIAN_POINT('Ctrl Pts',(0.85981294420286,-0.115492077056649,0.54708917182331));
#7944=CARTESIAN_POINT('Ctrl Pts',(0.850993704737257,-0.141695629206859,
0.560922177770136));
#7945=CARTESIAN_POINT('Ctrl Pts',(0.830754510485543,-0.181890537957859,
0.590422647829571));
#7946=CARTESIAN_POINT('Ctrl Pts',(0.816896541396381,-0.201072148666545,
0.609616703125488));
#7947=CARTESIAN_POINT('Ctrl Pts',(0.792310597819928,-0.223955109275652,
0.641117951819998));
#7948=CARTESIAN_POINT('Ctrl Pts',(0.779109323683612,-0.232742381310829,
0.657208095763053));
#7949=CARTESIAN_POINT('Ctrl Pts',(0.750552691816206,-0.244234834628584,
0.68964083160521));
#7950=CARTESIAN_POINT('Ctrl Pts',(0.735185187071673,-0.246942143572133,
0.705971972091755));
#7951=CARTESIAN_POINT('Ctrl Pts',(0.705971972091754,-0.246942143572133,
0.735185187071673));
#7952=CARTESIAN_POINT('Ctrl Pts',(0.689640831605209,-0.244234834628584,
0.750552691816206));
#7953=CARTESIAN_POINT('Ctrl Pts',(0.657208095763052,-0.232742381310829,
0.779109323683612));
#7954=CARTESIAN_POINT('Ctrl Pts',(0.641117951819998,-0.223955109275652,
0.792310597819928));
#7955=CARTESIAN_POINT('Ctrl Pts',(0.609616703125487,-0.201072148666545,
0.816896541396382));
#7956=CARTESIAN_POINT('Ctrl Pts',(0.590422647829571,-0.181890537957858,
0.830754510485544));
#7957=CARTESIAN_POINT('Ctrl Pts',(0.560922177770135,-0.141695629206858,
0.850993704737257));
#7958=CARTESIAN_POINT('Ctrl Pts',(0.547089171823309,-0.115492077056649,
0.859812944202861));
#7959=CARTESIAN_POINT('Ctrl Pts',(0.533674141594226,-0.0742967091364491,
0.868149331745852));
#7960=CARTESIAN_POINT('Ctrl Pts',(0.530395067942936,-0.0609922781173483,
0.870146645090731));
#7961=CARTESIAN_POINT('Ctrl Pts',(0.528110872004958,-0.0476300000000001,
0.871530771444223));
#7962=CARTESIAN_POINT('Origin',(0.707106781186547,-0.04763,0.707106781186548));
#7963=CARTESIAN_POINT('Origin',(0.,-0.166705,0.));
#7964=CARTESIAN_POINT('',(0.242834539687906,-0.04763,0.989696097314));
#7965=CARTESIAN_POINT('Origin',(0.,-0.04763,0.));
#7966=CARTESIAN_POINT('',(-0.242834539687907,-0.04763,0.989696097314));
#7967=CARTESIAN_POINT('Ctrl Pts',(0.242834539687906,-0.04763,0.989696097314));
#7968=CARTESIAN_POINT('Ctrl Pts',(0.24024064412003,-0.0609922781173483,
0.990332542620729));
#7969=CARTESIAN_POINT('Ctrl Pts',(0.236509675094874,-0.0742967091364492,
0.991238884025248));
#7970=CARTESIAN_POINT('Ctrl Pts',(0.221129100087819,-0.115492077056649,
0.994830026707808));
#7971=CARTESIAN_POINT('Ctrl Pts',(0.205111543747588,-0.141695629206859,
0.998375294985966));
#7972=CARTESIAN_POINT('Ctrl Pts',(0.169940289819232,-0.181890537957859,
1.00492400591205));
#7973=CARTESIAN_POINT('Ctrl Pts',(0.1465689792446,-0.201072148666545,1.00869718865384));
#7974=CARTESIAN_POINT('Ctrl Pts',(0.106909345252087,-0.223955109275652,
1.01358704779679));
#7975=CARTESIAN_POINT('Ctrl Pts',(0.0861971848975941,-0.232742381310829,
1.0156297872271));
#7976=CARTESIAN_POINT('Ctrl Pts',(0.0430711894098822,-0.244234834628584,
1.01837060663223));
#7977=CARTESIAN_POINT('Ctrl Pts',(0.0206568624125605,-0.246942143572133,
1.019052));
#7978=CARTESIAN_POINT('Ctrl Pts',(-0.0206568624125608,-0.246942143572133,
1.019052));
#7979=CARTESIAN_POINT('Ctrl Pts',(-0.0430711894098825,-0.244234834628584,
1.01837060663223));
#7980=CARTESIAN_POINT('Ctrl Pts',(-0.0861971848975943,-0.232742381310829,
1.0156297872271));
#7981=CARTESIAN_POINT('Ctrl Pts',(-0.106909345252088,-0.223955109275652,
1.01358704779679));
#7982=CARTESIAN_POINT('Ctrl Pts',(-0.1465689792446,-0.201072148666545,1.00869718865384));
#7983=CARTESIAN_POINT('Ctrl Pts',(-0.169940289819232,-0.181890537957859,
1.00492400591205));
#7984=CARTESIAN_POINT('Ctrl Pts',(-0.205111543747588,-0.141695629206859,
0.998375294985966));
#7985=CARTESIAN_POINT('Ctrl Pts',(-0.221129100087819,-0.115492077056649,
0.994830026707808));
#7986=CARTESIAN_POINT('Ctrl Pts',(-0.236509675094875,-0.0742967091364493,
0.991238884025248));
#7987=CARTESIAN_POINT('Ctrl Pts',(-0.24024064412003,-0.0609922781173483,
0.990332542620729));
#7988=CARTESIAN_POINT('Ctrl Pts',(-0.242834539687907,-0.04763,0.989696097314));
#7989=CARTESIAN_POINT('',(-0.528110872004959,-0.04763,0.871530771444223));
#7990=CARTESIAN_POINT('Origin',(0.,-0.04763,0.));
#7991=CARTESIAN_POINT('',(-0.871530771444223,-0.04763,0.528110872004958));
#7992=CARTESIAN_POINT('Ctrl Pts',(-0.528110872004958,-0.0476300000000001,
0.871530771444223));
#7993=CARTESIAN_POINT('Ctrl Pts',(-0.530395067942936,-0.0609922781173484,
0.87014664509073));
#7994=CARTESIAN_POINT('Ctrl Pts',(-0.533674141594226,-0.0742967091364493,
0.868149331745851));
#7995=CARTESIAN_POINT('Ctrl Pts',(-0.54708917182331,-0.115492077056649,
0.85981294420286));
#7996=CARTESIAN_POINT('Ctrl Pts',(-0.560922177770136,-0.141695629206859,
0.850993704737257));
#7997=CARTESIAN_POINT('Ctrl Pts',(-0.590422647829571,-0.181890537957859,
0.830754510485543));
#7998=CARTESIAN_POINT('Ctrl Pts',(-0.609616703125488,-0.201072148666545,
0.816896541396381));
#7999=CARTESIAN_POINT('Ctrl Pts',(-0.641117951819998,-0.223955109275652,
0.792310597819928));
#8000=CARTESIAN_POINT('Ctrl Pts',(-0.657208095763053,-0.232742381310829,
0.779109323683611));
#8001=CARTESIAN_POINT('Ctrl Pts',(-0.68964083160521,-0.244234834628584,
0.750552691816205));
#8002=CARTESIAN_POINT('Ctrl Pts',(-0.705971972091755,-0.246942143572133,
0.735185187071673));
#8003=CARTESIAN_POINT('Ctrl Pts',(-0.735185187071673,-0.246942143572133,
0.705971972091754));
#8004=CARTESIAN_POINT('Ctrl Pts',(-0.750552691816206,-0.244234834628584,
0.689640831605209));
#8005=CARTESIAN_POINT('Ctrl Pts',(-0.779109323683612,-0.232742381310829,
0.657208095763052));
#8006=CARTESIAN_POINT('Ctrl Pts',(-0.792310597819928,-0.223955109275652,
0.641117951819998));
#8007=CARTESIAN_POINT('Ctrl Pts',(-0.816896541396382,-0.201072148666545,
0.609616703125487));
#8008=CARTESIAN_POINT('Ctrl Pts',(-0.830754510485544,-0.181890537957858,
0.590422647829571));
#8009=CARTESIAN_POINT('Ctrl Pts',(-0.850993704737257,-0.141695629206858,
0.560922177770135));
#8010=CARTESIAN_POINT('Ctrl Pts',(-0.859812944202861,-0.115492077056649,
0.547089171823309));
#8011=CARTESIAN_POINT('Ctrl Pts',(-0.868149331745852,-0.0742967091364491,
0.533674141594226));
#8012=CARTESIAN_POINT('Ctrl Pts',(-0.870146645090731,-0.0609922781173483,
0.530395067942936));
#8013=CARTESIAN_POINT('Ctrl Pts',(-0.871530771444223,-0.04763,0.528110872004958));
#8014=CARTESIAN_POINT('',(-0.989696097314,-0.04763,0.242834539687906));
#8015=CARTESIAN_POINT('Origin',(0.,-0.04763,0.));
#8016=CARTESIAN_POINT('',(-1.019052,-0.246942143572133,1.248489836334E-16));
#8017=CARTESIAN_POINT('Ctrl Pts',(-0.989696097314,-0.04763,0.242834539687906));
#8018=CARTESIAN_POINT('Ctrl Pts',(-0.990332542620729,-0.0609922781173483,
0.24024064412003));
#8019=CARTESIAN_POINT('Ctrl Pts',(-0.991238884025248,-0.0742967091364492,
0.236509675094874));
#8020=CARTESIAN_POINT('Ctrl Pts',(-0.994830026707808,-0.115492077056649,
0.221129100087819));
#8021=CARTESIAN_POINT('Ctrl Pts',(-0.998375294985966,-0.141695629206859,
0.205111543747588));
#8022=CARTESIAN_POINT('Ctrl Pts',(-1.00492400591205,-0.181890537957859,
0.169940289819232));
#8023=CARTESIAN_POINT('Ctrl Pts',(-1.00869718865384,-0.201072148666545,
0.1465689792446));
#8024=CARTESIAN_POINT('Ctrl Pts',(-1.01358704779679,-0.223955109275652,
0.106909345252088));
#8025=CARTESIAN_POINT('Ctrl Pts',(-1.0156297872271,-0.232742381310829,0.0861971848975944));
#8026=CARTESIAN_POINT('Ctrl Pts',(-1.01837060663223,-0.244234834628584,
0.0430711894098825));
#8027=CARTESIAN_POINT('Ctrl Pts',(-1.019052,-0.246942143572133,0.0206568624125608));
#8028=CARTESIAN_POINT('Ctrl Pts',(-1.019052,-0.246942143572133,1.2490009027033E-16));
#8029=CARTESIAN_POINT('',(-1.019052,-0.28578,1.24797876996471E-16));
#8030=CARTESIAN_POINT('',(-1.019052,-0.166705,1.24797876996471E-16));
#8031=CARTESIAN_POINT('Origin',(0.,-0.28578,0.));
#8032=CARTESIAN_POINT('',(-0.989696097314,-0.04763,-0.242834539687906));
#8033=CARTESIAN_POINT('Ctrl Pts',(-1.019052,-0.246942143572133,1.2490009027033E-16));
#8034=CARTESIAN_POINT('Ctrl Pts',(-1.019052,-0.246942143572133,-0.0206568624125605));
#8035=CARTESIAN_POINT('Ctrl Pts',(-1.01837060663223,-0.244234834628584,
-0.0430711894098822));
#8036=CARTESIAN_POINT('Ctrl Pts',(-1.0156297872271,-0.232742381310829,-0.0861971848975941));
#8037=CARTESIAN_POINT('Ctrl Pts',(-1.01358704779679,-0.223955109275652,
-0.106909345252087));
#8038=CARTESIAN_POINT('Ctrl Pts',(-1.00869718865384,-0.201072148666546,
-0.1465689792446));
#8039=CARTESIAN_POINT('Ctrl Pts',(-1.00492400591205,-0.181890537957859,
-0.169940289819232));
#8040=CARTESIAN_POINT('Ctrl Pts',(-0.998375294985966,-0.141695629206859,
-0.205111543747588));
#8041=CARTESIAN_POINT('Ctrl Pts',(-0.994830026707808,-0.11549207705665,
-0.221129100087819));
#8042=CARTESIAN_POINT('Ctrl Pts',(-0.991238884025248,-0.0742967091364495,
-0.236509675094874));
#8043=CARTESIAN_POINT('Ctrl Pts',(-0.990332542620729,-0.0609922781173484,
-0.24024064412003));
#8044=CARTESIAN_POINT('Ctrl Pts',(-0.989696097314,-0.0476300000000001,-0.242834539687907));
#8045=CARTESIAN_POINT('',(-0.871530771444223,-0.04763,-0.528110872004958));
#8046=CARTESIAN_POINT('Origin',(0.,-0.04763,0.));
#8047=CARTESIAN_POINT('',(-0.528110872004958,-0.04763,-0.871530771444223));
#8048=CARTESIAN_POINT('Ctrl Pts',(-0.871530771444223,-0.0476300000000001,
-0.528110872004958));
#8049=CARTESIAN_POINT('Ctrl Pts',(-0.87014664509073,-0.0609922781173484,
-0.530395067942936));
#8050=CARTESIAN_POINT('Ctrl Pts',(-0.868149331745851,-0.0742967091364494,
-0.533674141594226));
#8051=CARTESIAN_POINT('Ctrl Pts',(-0.85981294420286,-0.115492077056649,
-0.54708917182331));
#8052=CARTESIAN_POINT('Ctrl Pts',(-0.850993704737257,-0.141695629206859,
-0.560922177770136));
#8053=CARTESIAN_POINT('Ctrl Pts',(-0.830754510485543,-0.181890537957859,
-0.590422647829571));
#8054=CARTESIAN_POINT('Ctrl Pts',(-0.816896541396381,-0.201072148666546,
-0.609616703125488));
#8055=CARTESIAN_POINT('Ctrl Pts',(-0.792310597819928,-0.223955109275652,
-0.641117951819999));
#8056=CARTESIAN_POINT('Ctrl Pts',(-0.779109323683611,-0.232742381310829,
-0.657208095763053));
#8057=CARTESIAN_POINT('Ctrl Pts',(-0.750552691816205,-0.244234834628584,
-0.68964083160521));
#8058=CARTESIAN_POINT('Ctrl Pts',(-0.735185187071673,-0.246942143572133,
-0.705971972091755));
#8059=CARTESIAN_POINT('Ctrl Pts',(-0.705971972091754,-0.246942143572133,
-0.735185187071673));
#8060=CARTESIAN_POINT('Ctrl Pts',(-0.68964083160521,-0.244234834628584,
-0.750552691816206));
#8061=CARTESIAN_POINT('Ctrl Pts',(-0.657208095763052,-0.232742381310829,
-0.779109323683612));
#8062=CARTESIAN_POINT('Ctrl Pts',(-0.641117951819998,-0.223955109275652,
-0.792310597819928));
#8063=CARTESIAN_POINT('Ctrl Pts',(-0.609616703125488,-0.201072148666545,
-0.816896541396381));
#8064=CARTESIAN_POINT('Ctrl Pts',(-0.590422647829571,-0.181890537957859,
-0.830754510485543));
#8065=CARTESIAN_POINT('Ctrl Pts',(-0.560922177770136,-0.141695629206859,
-0.850993704737257));
#8066=CARTESIAN_POINT('Ctrl Pts',(-0.54708917182331,-0.115492077056649,
-0.85981294420286));
#8067=CARTESIAN_POINT('Ctrl Pts',(-0.533674141594226,-0.0742967091364494,
-0.868149331745852));
#8068=CARTESIAN_POINT('Ctrl Pts',(-0.530395067942936,-0.0609922781173484,
-0.870146645090731));
#8069=CARTESIAN_POINT('Ctrl Pts',(-0.528110872004958,-0.0476300000000001,
-0.871530771444223));
#8070=CARTESIAN_POINT('',(-0.242834539687906,-0.04763,-0.989696097314));
#8071=CARTESIAN_POINT('Origin',(0.,-0.04763,0.));
#8072=CARTESIAN_POINT('',(0.242834539687906,-0.04763,-0.989696097314));
#8073=CARTESIAN_POINT('Ctrl Pts',(-0.242834539687907,-0.04763,-0.989696097314));
#8074=CARTESIAN_POINT('Ctrl Pts',(-0.24024064412003,-0.0609922781173483,
-0.990332542620729));
#8075=CARTESIAN_POINT('Ctrl Pts',(-0.236509675094874,-0.0742967091364493,
-0.991238884025248));
#8076=CARTESIAN_POINT('Ctrl Pts',(-0.221129100087819,-0.115492077056649,
-0.994830026707808));
#8077=CARTESIAN_POINT('Ctrl Pts',(-0.205111543747588,-0.141695629206859,
-0.998375294985966));
#8078=CARTESIAN_POINT('Ctrl Pts',(-0.169940289819232,-0.181890537957859,
-1.00492400591205));
#8079=CARTESIAN_POINT('Ctrl Pts',(-0.1465689792446,-0.201072148666545,-1.00869718865384));
#8080=CARTESIAN_POINT('Ctrl Pts',(-0.106909345252087,-0.223955109275652,
-1.01358704779679));
#8081=CARTESIAN_POINT('Ctrl Pts',(-0.0861971848975942,-0.232742381310829,
-1.0156297872271));
#8082=CARTESIAN_POINT('Ctrl Pts',(-0.0430711894098823,-0.244234834628584,
-1.01837060663223));
#8083=CARTESIAN_POINT('Ctrl Pts',(-0.0206568624125606,-0.246942143572133,
-1.019052));
#8084=CARTESIAN_POINT('Ctrl Pts',(0.0206568624125607,-0.246942143572133,
-1.019052));
#8085=CARTESIAN_POINT('Ctrl Pts',(0.0430711894098824,-0.244234834628584,
-1.01837060663223));
#8086=CARTESIAN_POINT('Ctrl Pts',(0.0861971848975943,-0.232742381310829,
-1.0156297872271));
#8087=CARTESIAN_POINT('Ctrl Pts',(0.106909345252088,-0.223955109275652,
-1.01358704779679));
#8088=CARTESIAN_POINT('Ctrl Pts',(0.1465689792446,-0.201072148666545,-1.00869718865384));
#8089=CARTESIAN_POINT('Ctrl Pts',(0.169940289819232,-0.181890537957859,
-1.00492400591205));
#8090=CARTESIAN_POINT('Ctrl Pts',(0.205111543747588,-0.141695629206859,
-0.998375294985966));
#8091=CARTESIAN_POINT('Ctrl Pts',(0.221129100087819,-0.115492077056649,
-0.994830026707808));
#8092=CARTESIAN_POINT('Ctrl Pts',(0.236509675094874,-0.0742967091364493,
-0.991238884025248));
#8093=CARTESIAN_POINT('Ctrl Pts',(0.24024064412003,-0.0609922781173484,
-0.990332542620729));
#8094=CARTESIAN_POINT('Ctrl Pts',(0.242834539687907,-0.04763,-0.989696097314));
#8095=CARTESIAN_POINT('',(0.528110872004958,-0.04763,-0.871530771444223));
#8096=CARTESIAN_POINT('Origin',(0.,-0.04763,0.));
#8097=CARTESIAN_POINT('',(0.871530771444223,-0.04763,-0.528110872004958));
#8098=CARTESIAN_POINT('Ctrl Pts',(0.528110872004958,-0.0476300000000001,
-0.871530771444223));
#8099=CARTESIAN_POINT('Ctrl Pts',(0.530395067942936,-0.0609922781173484,
-0.870146645090731));
#8100=CARTESIAN_POINT('Ctrl Pts',(0.533674141594226,-0.0742967091364493,
-0.868149331745851));
#8101=CARTESIAN_POINT('Ctrl Pts',(0.54708917182331,-0.115492077056649,-0.85981294420286));
#8102=CARTESIAN_POINT('Ctrl Pts',(0.560922177770136,-0.141695629206859,
-0.850993704737257));
#8103=CARTESIAN_POINT('Ctrl Pts',(0.590422647829571,-0.181890537957859,
-0.830754510485543));
#8104=CARTESIAN_POINT('Ctrl Pts',(0.609616703125488,-0.201072148666545,
-0.816896541396381));
#8105=CARTESIAN_POINT('Ctrl Pts',(0.641117951819998,-0.223955109275652,
-0.792310597819928));
#8106=CARTESIAN_POINT('Ctrl Pts',(0.657208095763053,-0.232742381310829,
-0.779109323683612));
#8107=CARTESIAN_POINT('Ctrl Pts',(0.68964083160521,-0.244234834628584,-0.750552691816206));
#8108=CARTESIAN_POINT('Ctrl Pts',(0.705971972091755,-0.246942143572133,
-0.735185187071673));
#8109=CARTESIAN_POINT('Ctrl Pts',(0.735185187071673,-0.246942143572133,
-0.705971972091754));
#8110=CARTESIAN_POINT('Ctrl Pts',(0.750552691816206,-0.244234834628584,
-0.68964083160521));
#8111=CARTESIAN_POINT('Ctrl Pts',(0.779109323683612,-0.232742381310829,
-0.657208095763053));
#8112=CARTESIAN_POINT('Ctrl Pts',(0.792310597819928,-0.223955109275652,
-0.641117951819998));
#8113=CARTESIAN_POINT('Ctrl Pts',(0.816896541396381,-0.201072148666545,
-0.609616703125488));
#8114=CARTESIAN_POINT('Ctrl Pts',(0.830754510485543,-0.181890537957859,
-0.590422647829571));
#8115=CARTESIAN_POINT('Ctrl Pts',(0.850993704737257,-0.141695629206859,
-0.560922177770136));
#8116=CARTESIAN_POINT('Ctrl Pts',(0.85981294420286,-0.115492077056649,-0.54708917182331));
#8117=CARTESIAN_POINT('Ctrl Pts',(0.868149331745851,-0.0742967091364493,
-0.533674141594226));
#8118=CARTESIAN_POINT('Ctrl Pts',(0.870146645090731,-0.0609922781173484,
-0.530395067942936));
#8119=CARTESIAN_POINT('Ctrl Pts',(0.871530771444223,-0.0476300000000001,
-0.528110872004958));
#8120=CARTESIAN_POINT('',(0.989696097314,-0.04763,-0.242834539687906));
#8121=CARTESIAN_POINT('Origin',(0.,-0.04763,0.));
#8122=CARTESIAN_POINT('',(0.989696097314,-0.04763,0.242834539687906));
#8123=CARTESIAN_POINT('Ctrl Pts',(0.989696097314,-0.04763,-0.242834539687907));
#8124=CARTESIAN_POINT('Ctrl Pts',(0.990332542620729,-0.0609922781173483,
-0.24024064412003));
#8125=CARTESIAN_POINT('Ctrl Pts',(0.991238884025248,-0.0742967091364493,
-0.236509675094874));
#8126=CARTESIAN_POINT('Ctrl Pts',(0.994830026707808,-0.115492077056649,
-0.221129100087819));
#8127=CARTESIAN_POINT('Ctrl Pts',(0.998375294985966,-0.141695629206859,
-0.205111543747588));
#8128=CARTESIAN_POINT('Ctrl Pts',(1.00492400591205,-0.181890537957859,-0.169940289819232));
#8129=CARTESIAN_POINT('Ctrl Pts',(1.00869718865384,-0.201072148666545,-0.1465689792446));
#8130=CARTESIAN_POINT('Ctrl Pts',(1.01358704779679,-0.223955109275652,-0.106909345252087));
#8131=CARTESIAN_POINT('Ctrl Pts',(1.0156297872271,-0.232742381310829,-0.0861971848975942));
#8132=CARTESIAN_POINT('Ctrl Pts',(1.01837060663223,-0.244234834628584,-0.0430711894098823));
#8133=CARTESIAN_POINT('Ctrl Pts',(1.019052,-0.246942143572133,-0.0206568624125607));
#8134=CARTESIAN_POINT('Ctrl Pts',(1.019052,-0.246942143572133,0.0206568624125607));
#8135=CARTESIAN_POINT('Ctrl Pts',(1.01837060663223,-0.244234834628584,0.0430711894098823));
#8136=CARTESIAN_POINT('Ctrl Pts',(1.0156297872271,-0.232742381310829,0.0861971848975942));
#8137=CARTESIAN_POINT('Ctrl Pts',(1.01358704779679,-0.223955109275652,0.106909345252087));
#8138=CARTESIAN_POINT('Ctrl Pts',(1.00869718865384,-0.201072148666545,0.1465689792446));
#8139=CARTESIAN_POINT('Ctrl Pts',(1.00492400591205,-0.181890537957859,0.169940289819232));
#8140=CARTESIAN_POINT('Ctrl Pts',(0.998375294985966,-0.141695629206859,
0.205111543747588));
#8141=CARTESIAN_POINT('Ctrl Pts',(0.994830026707808,-0.115492077056649,
0.221129100087819));
#8142=CARTESIAN_POINT('Ctrl Pts',(0.991238884025248,-0.0742967091364492,
0.236509675094874));
#8143=CARTESIAN_POINT('Ctrl Pts',(0.990332542620729,-0.0609922781173483,
0.24024064412003));
#8144=CARTESIAN_POINT('Ctrl Pts',(0.989696097314,-0.04763,0.242834539687907));
#8145=CARTESIAN_POINT('Origin',(0.,-0.04763,0.));
#8146=CARTESIAN_POINT('Origin',(0.,-0.04763,0.));
#8147=CARTESIAN_POINT('',(0.238183666596899,-0.04763,0.951592097314));
#8148=CARTESIAN_POINT('Origin',(0.,-0.04763,0.));
#8149=CARTESIAN_POINT('Origin',(-1.94289029309402E-16,-0.04763,1.));
#8150=CARTESIAN_POINT('Origin',(-1.94289029309402E-16,0.,1.));
#8151=CARTESIAN_POINT('',(-0.2381836665969,-0.04763,0.951592097314));
#8152=CARTESIAN_POINT('Ctrl Pts',(-0.238183666596899,-0.0476299999999999,
0.951592097314));
#8153=CARTESIAN_POINT('Ctrl Pts',(-0.233157223576062,-0.0740444353928835,
0.952850216871763));
#8154=CARTESIAN_POINT('Ctrl Pts',(-0.223801617934946,-0.0999305678883309,
0.955173119738174));
#8155=CARTESIAN_POINT('Ctrl Pts',(-0.199966927975188,-0.142345102874864,
0.960411259488514));
#8156=CARTESIAN_POINT('Ctrl Pts',(-0.1868781821531,-0.159766064500479,0.963103647174702));
#8157=CARTESIAN_POINT('Ctrl Pts',(-0.15681442133453,-0.190326085855194,
0.968453058988463));
#8158=CARTESIAN_POINT('Ctrl Pts',(-0.139836317888043,-0.203463743702801,
0.971100730005489));
#8159=CARTESIAN_POINT('Ctrl Pts',(-0.104422493053067,-0.224161999508995,
0.975530745318961));
#8160=CARTESIAN_POINT('Ctrl Pts',(-0.0842175114474176,-0.232861760990032,
0.977553872336861));
#8161=CARTESIAN_POINT('Ctrl Pts',(-0.0421062857595701,-0.244251601209411,
0.980270995488453));
#8162=CARTESIAN_POINT('Ctrl Pts',(-0.0201990724523197,-0.246942143572133,
0.980948));
#8163=CARTESIAN_POINT('Ctrl Pts',(0.020199072452319,-0.246942143572133,
0.980948));
#8164=CARTESIAN_POINT('Ctrl Pts',(0.0421062857595694,-0.244251601209411,
0.980270995488454));
#8165=CARTESIAN_POINT('Ctrl Pts',(0.0842175114474169,-0.232861760990032,
0.977553872336861));
#8166=CARTESIAN_POINT('Ctrl Pts',(0.104422493053067,-0.224161999508995,
0.975530745318961));
#8167=CARTESIAN_POINT('Ctrl Pts',(0.139836317888042,-0.203463743702801,
0.971100730005489));
#8168=CARTESIAN_POINT('Ctrl Pts',(0.15681442133453,-0.190326085855194,0.968453058988463));
#8169=CARTESIAN_POINT('Ctrl Pts',(0.1868781821531,-0.15976606450048,0.963103647174702));
#8170=CARTESIAN_POINT('Ctrl Pts',(0.199966927975188,-0.142345102874864,
0.960411259488514));
#8171=CARTESIAN_POINT('Ctrl Pts',(0.223801617934945,-0.0999305678883309,
0.955173119738174));
#8172=CARTESIAN_POINT('Ctrl Pts',(0.233157223576061,-0.0740444353928835,
0.952850216871763));
#8173=CARTESIAN_POINT('Ctrl Pts',(0.238183666596899,-0.0476299999999999,
0.951592097314));
#8174=CARTESIAN_POINT('Origin',(-1.94289029309402E-16,-0.04763,1.));
#8175=CARTESIAN_POINT('Origin',(0.,-0.04763,0.));
#8176=CARTESIAN_POINT('',(-0.504455939115715,-0.04763,0.841298510752802));
#8177=CARTESIAN_POINT('Origin',(0.,-0.04763,0.));
#8178=CARTESIAN_POINT('Origin',(-0.707106781186548,-0.04763,0.707106781186547));
#8179=CARTESIAN_POINT('Origin',(-0.707106781186548,0.,0.707106781186547));
#8180=CARTESIAN_POINT('',(-0.841298510752802,-0.04763,0.504455939115715));
#8181=CARTESIAN_POINT('Ctrl Pts',(-0.841298510752802,-0.04763,0.504455939115715));
#8182=CARTESIAN_POINT('Ctrl Pts',(-0.838633903678357,-0.0740444353928835,
0.508899795931835));
#8183=CARTESIAN_POINT('Ctrl Pts',(-0.833661031856294,-0.0999305678883309,
0.517157748491652));
#8184=CARTESIAN_POINT('Ctrl Pts',(-0.820511285096538,-0.142345102874864,
0.537715343527944));
#8185=CARTESIAN_POINT('Ctrl Pts',(-0.813159949759,-0.159766064500479,0.548874290046456));
#8186=CARTESIAN_POINT('Ctrl Pts',(-0.795684265985089,-0.190326085855194,
0.573915184558107));
#8187=CARTESIAN_POINT('Ctrl Pts',(-0.78555112003688,-0.203463743702801,
0.587792702767295));
#8188=CARTESIAN_POINT('Ctrl Pts',(-0.763642258217233,-0.224161999508995,
0.615966552324775));
#8189=CARTESIAN_POINT('Ctrl Pts',(-0.750785745543687,-0.232861760990032,
0.631684198665438));
#8190=CARTESIAN_POINT('Ctrl Pts',(-0.722929908501543,-0.244251601209411,
0.663382628119203));
#8191=CARTESIAN_POINT('Ctrl Pts',(-0.707917883896095,-0.246942143572133,
0.679352081686668));
#8192=CARTESIAN_POINT('Ctrl Pts',(-0.679352081686668,-0.246942143572133,
0.707917883896095));
#8193=CARTESIAN_POINT('Ctrl Pts',(-0.663382628119203,-0.244251601209411,
0.722929908501544));
#8194=CARTESIAN_POINT('Ctrl Pts',(-0.631684198665438,-0.232861760990031,
0.750785745543687));
#8195=CARTESIAN_POINT('Ctrl Pts',(-0.615966552324775,-0.224161999508995,
0.763642258217233));
#8196=CARTESIAN_POINT('Ctrl Pts',(-0.587792702767295,-0.203463743702801,
0.78555112003688));
#8197=CARTESIAN_POINT('Ctrl Pts',(-0.573915184558107,-0.190326085855194,
0.795684265985088));
#8198=CARTESIAN_POINT('Ctrl Pts',(-0.548874290046456,-0.159766064500479,
0.813159949759));
#8199=CARTESIAN_POINT('Ctrl Pts',(-0.537715343527944,-0.142345102874864,
0.820511285096538));
#8200=CARTESIAN_POINT('Ctrl Pts',(-0.517157748491652,-0.0999305678883309,
0.833661031856294));
#8201=CARTESIAN_POINT('Ctrl Pts',(-0.508899795931835,-0.0740444353928835,
0.838633903678357));
#8202=CARTESIAN_POINT('Ctrl Pts',(-0.504455939115716,-0.04763,0.841298510752801));
#8203=CARTESIAN_POINT('Origin',(-0.707106781186548,-0.04763,0.707106781186547));
#8204=CARTESIAN_POINT('Origin',(0.,-0.04763,0.));
#8205=CARTESIAN_POINT('',(-0.951592097314,-0.04763,0.238183666596899));
#8206=CARTESIAN_POINT('Origin',(0.,-0.04763,0.));
#8207=CARTESIAN_POINT('Origin',(-1.,-0.04763,-1.11022302462516E-16));
#8208=CARTESIAN_POINT('Origin',(-1.,0.,-1.11022302462516E-16));
#8209=CARTESIAN_POINT('',(-0.951592097314,-0.04763,-0.2381836665969));
#8210=CARTESIAN_POINT('',(-0.980948,-0.246942143572133,1.08514323328844E-18));
#8211=CARTESIAN_POINT('Ctrl Pts',(-0.951592097314,-0.04763,-0.238183666596899));
#8212=CARTESIAN_POINT('Ctrl Pts',(-0.952850216871763,-0.0740444353928835,
-0.233157223576062));
#8213=CARTESIAN_POINT('Ctrl Pts',(-0.955173119738174,-0.0999305678883309,
-0.223801617934946));
#8214=CARTESIAN_POINT('Ctrl Pts',(-0.960411259488514,-0.142345102874864,
-0.199966927975188));
#8215=CARTESIAN_POINT('Ctrl Pts',(-0.963103647174702,-0.159766064500479,
-0.1868781821531));
#8216=CARTESIAN_POINT('Ctrl Pts',(-0.968453058988463,-0.190326085855194,
-0.15681442133453));
#8217=CARTESIAN_POINT('Ctrl Pts',(-0.971100730005489,-0.203463743702801,
-0.139836317888043));
#8218=CARTESIAN_POINT('Ctrl Pts',(-0.975530745318961,-0.224161999508995,
-0.104422493053067));
#8219=CARTESIAN_POINT('Ctrl Pts',(-0.977553872336861,-0.232861760990032,
-0.0842175114474175));
#8220=CARTESIAN_POINT('Ctrl Pts',(-0.980270995488453,-0.244251601209411,
-0.0421062857595699));
#8221=CARTESIAN_POINT('Ctrl Pts',(-0.980948,-0.246942143572133,-0.0201990724523195));
#8222=CARTESIAN_POINT('Ctrl Pts',(-0.980948,-0.246942143572133,-1.17961196366423E-16));
#8223=CARTESIAN_POINT('Origin',(-1.,-0.04763,-1.11022302462516E-16));
#8224=CARTESIAN_POINT('Ctrl Pts',(-0.980948,-0.246942143572133,-1.17961196366423E-16));
#8225=CARTESIAN_POINT('Ctrl Pts',(-0.980948,-0.246942143572133,0.0201990724523192));
#8226=CARTESIAN_POINT('Ctrl Pts',(-0.980270995488453,-0.244251601209411,
0.0421062857595695));
#8227=CARTESIAN_POINT('Ctrl Pts',(-0.977553872336861,-0.232861760990032,
0.0842175114474169));
#8228=CARTESIAN_POINT('Ctrl Pts',(-0.975530745318961,-0.224161999508995,
0.104422493053066));
#8229=CARTESIAN_POINT('Ctrl Pts',(-0.971100730005489,-0.203463743702801,
0.139836317888042));
#8230=CARTESIAN_POINT('Ctrl Pts',(-0.968453058988463,-0.190326085855194,
0.15681442133453));
#8231=CARTESIAN_POINT('Ctrl Pts',(-0.963103647174702,-0.15976606450048,
0.1868781821531));
#8232=CARTESIAN_POINT('Ctrl Pts',(-0.960411259488514,-0.142345102874864,
0.199966927975188));
#8233=CARTESIAN_POINT('Ctrl Pts',(-0.955173119738174,-0.099930567888331,
0.223801617934945));
#8234=CARTESIAN_POINT('Ctrl Pts',(-0.952850216871763,-0.0740444353928835,
0.233157223576061));
#8235=CARTESIAN_POINT('Ctrl Pts',(-0.951592097314,-0.04763,0.238183666596899));
#8236=CARTESIAN_POINT('Origin',(0.,-0.04763,0.));
#8237=CARTESIAN_POINT('',(-0.841298510752802,-0.04763,-0.504455939115715));
#8238=CARTESIAN_POINT('Origin',(0.,-0.04763,0.));
#8239=CARTESIAN_POINT('Origin',(-0.707106781186547,-0.04763,-0.707106781186548));
#8240=CARTESIAN_POINT('Origin',(-0.707106781186547,0.,-0.707106781186548));
#8241=CARTESIAN_POINT('',(-0.504455939115715,-0.04763,-0.841298510752802));
#8242=CARTESIAN_POINT('Ctrl Pts',(-0.504455939115715,-0.04763,-0.841298510752802));
#8243=CARTESIAN_POINT('Ctrl Pts',(-0.508899795931835,-0.0740444353928835,
-0.838633903678357));
#8244=CARTESIAN_POINT('Ctrl Pts',(-0.517157748491652,-0.0999305678883309,
-0.833661031856294));
#8245=CARTESIAN_POINT('Ctrl Pts',(-0.537715343527944,-0.142345102874864,
-0.820511285096538));
#8246=CARTESIAN_POINT('Ctrl Pts',(-0.548874290046456,-0.159766064500479,
-0.813159949759));
#8247=CARTESIAN_POINT('Ctrl Pts',(-0.573915184558107,-0.190326085855194,
-0.795684265985089));
#8248=CARTESIAN_POINT('Ctrl Pts',(-0.587792702767295,-0.203463743702801,
-0.78555112003688));
#8249=CARTESIAN_POINT('Ctrl Pts',(-0.615966552324775,-0.224161999508995,
-0.763642258217233));
#8250=CARTESIAN_POINT('Ctrl Pts',(-0.631684198665438,-0.232861760990032,
-0.750785745543687));
#8251=CARTESIAN_POINT('Ctrl Pts',(-0.663382628119203,-0.244251601209411,
-0.722929908501543));
#8252=CARTESIAN_POINT('Ctrl Pts',(-0.679352081686668,-0.246942143572133,
-0.707917883896095));
#8253=CARTESIAN_POINT('Ctrl Pts',(-0.707917883896095,-0.246942143572133,
-0.679352081686668));
#8254=CARTESIAN_POINT('Ctrl Pts',(-0.722929908501543,-0.244251601209411,
-0.663382628119203));
#8255=CARTESIAN_POINT('Ctrl Pts',(-0.750785745543687,-0.232861760990032,
-0.631684198665439));
#8256=CARTESIAN_POINT('Ctrl Pts',(-0.763642258217232,-0.224161999508995,
-0.615966552324775));
#8257=CARTESIAN_POINT('Ctrl Pts',(-0.78555112003688,-0.203463743702801,
-0.587792702767295));
#8258=CARTESIAN_POINT('Ctrl Pts',(-0.795684265985088,-0.190326085855194,
-0.573915184558107));
#8259=CARTESIAN_POINT('Ctrl Pts',(-0.813159949759,-0.15976606450048,-0.548874290046456));
#8260=CARTESIAN_POINT('Ctrl Pts',(-0.820511285096538,-0.142345102874864,
-0.537715343527944));
#8261=CARTESIAN_POINT('Ctrl Pts',(-0.833661031856294,-0.0999305678883311,
-0.517157748491652));
#8262=CARTESIAN_POINT('Ctrl Pts',(-0.838633903678357,-0.0740444353928836,
-0.508899795931835));
#8263=CARTESIAN_POINT('Ctrl Pts',(-0.841298510752801,-0.04763,-0.504455939115715));
#8264=CARTESIAN_POINT('Origin',(-0.707106781186547,-0.04763,-0.707106781186548));
#8265=CARTESIAN_POINT('Origin',(0.,-0.04763,0.));
#8266=CARTESIAN_POINT('',(-0.238183666596899,-0.04763,-0.951592097314));
#8267=CARTESIAN_POINT('Origin',(0.,-0.04763,0.));
#8268=CARTESIAN_POINT('Origin',(5.55111512312578E-17,-0.04763,-1.));
#8269=CARTESIAN_POINT('Origin',(5.55111512312578E-17,0.,-1.));
#8270=CARTESIAN_POINT('',(0.238183666596899,-0.04763,-0.951592097314));
#8271=CARTESIAN_POINT('Ctrl Pts',(0.238183666596899,-0.04763,-0.951592097314));
#8272=CARTESIAN_POINT('Ctrl Pts',(0.233157223576062,-0.0740444353928835,
-0.952850216871763));
#8273=CARTESIAN_POINT('Ctrl Pts',(0.223801617934946,-0.099930567888331,
-0.955173119738174));
#8274=CARTESIAN_POINT('Ctrl Pts',(0.199966927975188,-0.142345102874864,
-0.960411259488514));
#8275=CARTESIAN_POINT('Ctrl Pts',(0.1868781821531,-0.15976606450048,-0.963103647174702));
#8276=CARTESIAN_POINT('Ctrl Pts',(0.15681442133453,-0.190326085855194,-0.968453058988463));
#8277=CARTESIAN_POINT('Ctrl Pts',(0.139836317888042,-0.203463743702801,
-0.971100730005489));
#8278=CARTESIAN_POINT('Ctrl Pts',(0.104422493053067,-0.224161999508995,
-0.975530745318961));
#8279=CARTESIAN_POINT('Ctrl Pts',(0.0842175114474173,-0.232861760990032,
-0.977553872336861));
#8280=CARTESIAN_POINT('Ctrl Pts',(0.0421062857595698,-0.244251601209411,
-0.980270995488453));
#8281=CARTESIAN_POINT('Ctrl Pts',(0.0201990724523194,-0.246942143572133,
-0.980948));
#8282=CARTESIAN_POINT('Ctrl Pts',(-0.0201990724523193,-0.246942143572133,
-0.980948));
#8283=CARTESIAN_POINT('Ctrl Pts',(-0.0421062857595697,-0.244251601209411,
-0.980270995488453));
#8284=CARTESIAN_POINT('Ctrl Pts',(-0.0842175114474171,-0.232861760990032,
-0.977553872336861));
#8285=CARTESIAN_POINT('Ctrl Pts',(-0.104422493053067,-0.224161999508995,
-0.975530745318961));
#8286=CARTESIAN_POINT('Ctrl Pts',(-0.139836317888042,-0.203463743702801,
-0.971100730005489));
#8287=CARTESIAN_POINT('Ctrl Pts',(-0.15681442133453,-0.190326085855194,
-0.968453058988463));
#8288=CARTESIAN_POINT('Ctrl Pts',(-0.1868781821531,-0.15976606450048,-0.963103647174702));
#8289=CARTESIAN_POINT('Ctrl Pts',(-0.199966927975188,-0.142345102874864,
-0.960411259488514));
#8290=CARTESIAN_POINT('Ctrl Pts',(-0.223801617934945,-0.099930567888331,
-0.955173119738174));
#8291=CARTESIAN_POINT('Ctrl Pts',(-0.233157223576062,-0.0740444353928835,
-0.952850216871763));
#8292=CARTESIAN_POINT('Ctrl Pts',(-0.238183666596899,-0.0476299999999999,
-0.951592097314));
#8293=CARTESIAN_POINT('Origin',(5.55111512312578E-17,-0.04763,-1.));
#8294=CARTESIAN_POINT('Origin',(0.,-0.04763,0.));
#8295=CARTESIAN_POINT('',(0.504455939115715,-0.04763,-0.841298510752802));
#8296=CARTESIAN_POINT('Origin',(0.,-0.04763,0.));
#8297=CARTESIAN_POINT('Origin',(0.707106781186548,-0.04763,-0.707106781186547));
#8298=CARTESIAN_POINT('Origin',(0.707106781186548,0.,-0.707106781186547));
#8299=CARTESIAN_POINT('',(0.841298510752802,-0.04763,-0.504455939115715));
#8300=CARTESIAN_POINT('Ctrl Pts',(0.841298510752802,-0.04763,-0.504455939115715));
#8301=CARTESIAN_POINT('Ctrl Pts',(0.838633903678357,-0.0740444353928835,
-0.508899795931835));
#8302=CARTESIAN_POINT('Ctrl Pts',(0.833661031856294,-0.0999305678883309,
-0.517157748491652));
#8303=CARTESIAN_POINT('Ctrl Pts',(0.820511285096538,-0.142345102874864,
-0.537715343527944));
#8304=CARTESIAN_POINT('Ctrl Pts',(0.813159949759,-0.159766064500479,-0.548874290046456));
#8305=CARTESIAN_POINT('Ctrl Pts',(0.795684265985088,-0.190326085855194,
-0.573915184558107));
#8306=CARTESIAN_POINT('Ctrl Pts',(0.78555112003688,-0.203463743702801,-0.587792702767295));
#8307=CARTESIAN_POINT('Ctrl Pts',(0.763642258217233,-0.224161999508995,
-0.615966552324775));
#8308=CARTESIAN_POINT('Ctrl Pts',(0.750785745543687,-0.232861760990032,
-0.631684198665438));
#8309=CARTESIAN_POINT('Ctrl Pts',(0.722929908501543,-0.244251601209411,
-0.663382628119203));
#8310=CARTESIAN_POINT('Ctrl Pts',(0.707917883896095,-0.246942143572133,
-0.679352081686668));
#8311=CARTESIAN_POINT('Ctrl Pts',(0.679352081686668,-0.246942143572133,
-0.707917883896095));
#8312=CARTESIAN_POINT('Ctrl Pts',(0.663382628119203,-0.244251601209411,
-0.722929908501543));
#8313=CARTESIAN_POINT('Ctrl Pts',(0.631684198665438,-0.232861760990032,
-0.750785745543687));
#8314=CARTESIAN_POINT('Ctrl Pts',(0.615966552324775,-0.224161999508995,
-0.763642258217232));
#8315=CARTESIAN_POINT('Ctrl Pts',(0.587792702767295,-0.203463743702801,
-0.78555112003688));
#8316=CARTESIAN_POINT('Ctrl Pts',(0.573915184558107,-0.190326085855194,
-0.795684265985088));
#8317=CARTESIAN_POINT('Ctrl Pts',(0.548874290046456,-0.159766064500479,
-0.813159949759));
#8318=CARTESIAN_POINT('Ctrl Pts',(0.537715343527944,-0.142345102874864,
-0.820511285096538));
#8319=CARTESIAN_POINT('Ctrl Pts',(0.517157748491652,-0.099930567888331,
-0.833661031856294));
#8320=CARTESIAN_POINT('Ctrl Pts',(0.508899795931835,-0.0740444353928835,
-0.838633903678357));
#8321=CARTESIAN_POINT('Ctrl Pts',(0.504455939115715,-0.04763,-0.841298510752801));
#8322=CARTESIAN_POINT('Origin',(0.707106781186548,-0.04763,-0.707106781186547));
#8323=CARTESIAN_POINT('Origin',(0.,-0.166705,0.));
#8324=CARTESIAN_POINT('',(-0.980948,-0.28578,1.20131482833E-16));
#8325=CARTESIAN_POINT('Origin',(0.,-0.28578,0.));
#8326=CARTESIAN_POINT('',(-0.980948,-0.166705,1.20131482833E-16));
#8327=CARTESIAN_POINT('',(0.951592097314,-0.04763,0.238183666596899));
#8328=CARTESIAN_POINT('Origin',(0.,-0.04763,0.));
#8329=CARTESIAN_POINT('',(0.951592097314,-0.04763,-0.238183666596899));
#8330=CARTESIAN_POINT('Ctrl Pts',(0.951592097314,-0.04763,0.238183666596899));
#8331=CARTESIAN_POINT('Ctrl Pts',(0.952850216871763,-0.0740444353928835,
0.233157223576062));
#8332=CARTESIAN_POINT('Ctrl Pts',(0.955173119738174,-0.099930567888331,
0.223801617934945));
#8333=CARTESIAN_POINT('Ctrl Pts',(0.960411259488514,-0.142345102874864,
0.199966927975188));
#8334=CARTESIAN_POINT('Ctrl Pts',(0.963103647174702,-0.15976606450048,0.1868781821531));
#8335=CARTESIAN_POINT('Ctrl Pts',(0.968453058988463,-0.190326085855194,
0.15681442133453));
#8336=CARTESIAN_POINT('Ctrl Pts',(0.971100730005489,-0.203463743702801,
0.139836317888042));
#8337=CARTESIAN_POINT('Ctrl Pts',(0.975530745318961,-0.224161999508995,
0.104422493053067));
#8338=CARTESIAN_POINT('Ctrl Pts',(0.977553872336861,-0.232861760990032,
0.0842175114474172));
#8339=CARTESIAN_POINT('Ctrl Pts',(0.980270995488453,-0.244251601209411,
0.0421062857595697));
#8340=CARTESIAN_POINT('Ctrl Pts',(0.980948,-0.246942143572133,0.0201990724523194));
#8341=CARTESIAN_POINT('Ctrl Pts',(0.980948,-0.246942143572133,-0.0201990724523194));
#8342=CARTESIAN_POINT('Ctrl Pts',(0.980270995488453,-0.244251601209411,
-0.0421062857595697));
#8343=CARTESIAN_POINT('Ctrl Pts',(0.977553872336861,-0.232861760990032,
-0.0842175114474172));
#8344=CARTESIAN_POINT('Ctrl Pts',(0.975530745318961,-0.224161999508995,
-0.104422493053067));
#8345=CARTESIAN_POINT('Ctrl Pts',(0.971100730005489,-0.203463743702801,
-0.139836317888042));
#8346=CARTESIAN_POINT('Ctrl Pts',(0.968453058988463,-0.190326085855194,
-0.15681442133453));
#8347=CARTESIAN_POINT('Ctrl Pts',(0.963103647174702,-0.15976606450048,-0.1868781821531));
#8348=CARTESIAN_POINT('Ctrl Pts',(0.960411259488514,-0.142345102874864,
-0.199966927975188));
#8349=CARTESIAN_POINT('Ctrl Pts',(0.955173119738174,-0.099930567888331,
-0.223801617934945));
#8350=CARTESIAN_POINT('Ctrl Pts',(0.952850216871763,-0.0740444353928835,
-0.233157223576062));
#8351=CARTESIAN_POINT('Ctrl Pts',(0.951592097314,-0.0476299999999999,-0.238183666596899));
#8352=CARTESIAN_POINT('Origin',(0.,-0.04763,0.));
#8353=CARTESIAN_POINT('Origin',(0.,-0.04763,0.));
#8354=CARTESIAN_POINT('Origin',(1.,-0.04763,0.));
#8355=CARTESIAN_POINT('Origin',(1.,0.,0.));
#8356=CARTESIAN_POINT('Origin',(1.,-0.04763,0.));
#8357=CARTESIAN_POINT('Origin',(0.,-0.28578,0.));
#8358=CARTESIAN_POINT('Origin',(0.,-0.04763,0.));
#9574=UNCERTAINTY_MEASURE_WITH_UNIT(LENGTH_MEASURE(0.001),#9623,
'DISTANCE_ACCURACY_VALUE',
'Maximum model space distance between geometric entities at asserted c
onnectivities');
#9592=UNCERTAINTY_MEASURE_WITH_UNIT(LENGTH_MEASURE(0.001),#9623,
'DISTANCE_ACCURACY_VALUE',
'Maximum model space distance between geometric entities at asserted c
onnectivities');
#9604=(
GEOMETRIC_REPRESENTATION_CONTEXT(3)
GLOBAL_UNCERTAINTY_ASSIGNED_CONTEXT((#9574))
GLOBAL_UNIT_ASSIGNED_CONTEXT((#9623,#9625,#9626))
REPRESENTATION_CONTEXT('','3D')
);
#9622=(
GEOMETRIC_REPRESENTATION_CONTEXT(3)
GLOBAL_UNCERTAINTY_ASSIGNED_CONTEXT((#9592))
GLOBAL_UNIT_ASSIGNED_CONTEXT((#9623,#9625,#9626))
REPRESENTATION_CONTEXT('','3D')
);
#9623=(
LENGTH_UNIT()
NAMED_UNIT(*)
SI_UNIT(.CENTI.,.METRE.)
);
#9625=(
NAMED_UNIT(*)
PLANE_ANGLE_UNIT()
SI_UNIT($,.RADIAN.)
);
#9626=(
NAMED_UNIT(*)
SI_UNIT($,.STERADIAN.)
SOLID_ANGLE_UNIT()
);
#9638=SHAPE_DEFINITION_REPRESENTATION(#9667,#9755);
#9667=PRODUCT_DEFINITION_SHAPE('',$,#9785);
#9755=SHAPE_REPRESENTATION('',(#5627),#9604);
#9773=PRODUCT_DEFINITION_CONTEXT('part definition',#9862,'design');
#9785=PRODUCT_DEFINITION('Cage','Cage',#9814,#9773);
#9814=PRODUCT_DEFINITION_FORMATION('',$,#9875);
#9862=APPLICATION_CONTEXT(
'Core Data for Automotive Mechanical Design Process');
#9863=PRODUCT_CONTEXT('part definition',#9862,'mechanical');
#9875=PRODUCT('Cage','Cage','Cage',(#9863));
#9956=COLOUR_RGB('Grey',0.48,0.52,0.57);
#9957=FILL_AREA_STYLE_COLOUR('',#9956);
#9958=FILL_AREA_STYLE('',(#9957));
#9959=SURFACE_STYLE_FILL_AREA(#9958);
#9960=SURFACE_SIDE_STYLE('',(#9959));
#9961=SURFACE_STYLE_USAGE(.BOTH.,#9960);
#9962=PRESENTATION_STYLE_ASSIGNMENT((#9961));
ENDSEC;
END-ISO-10303-21;
